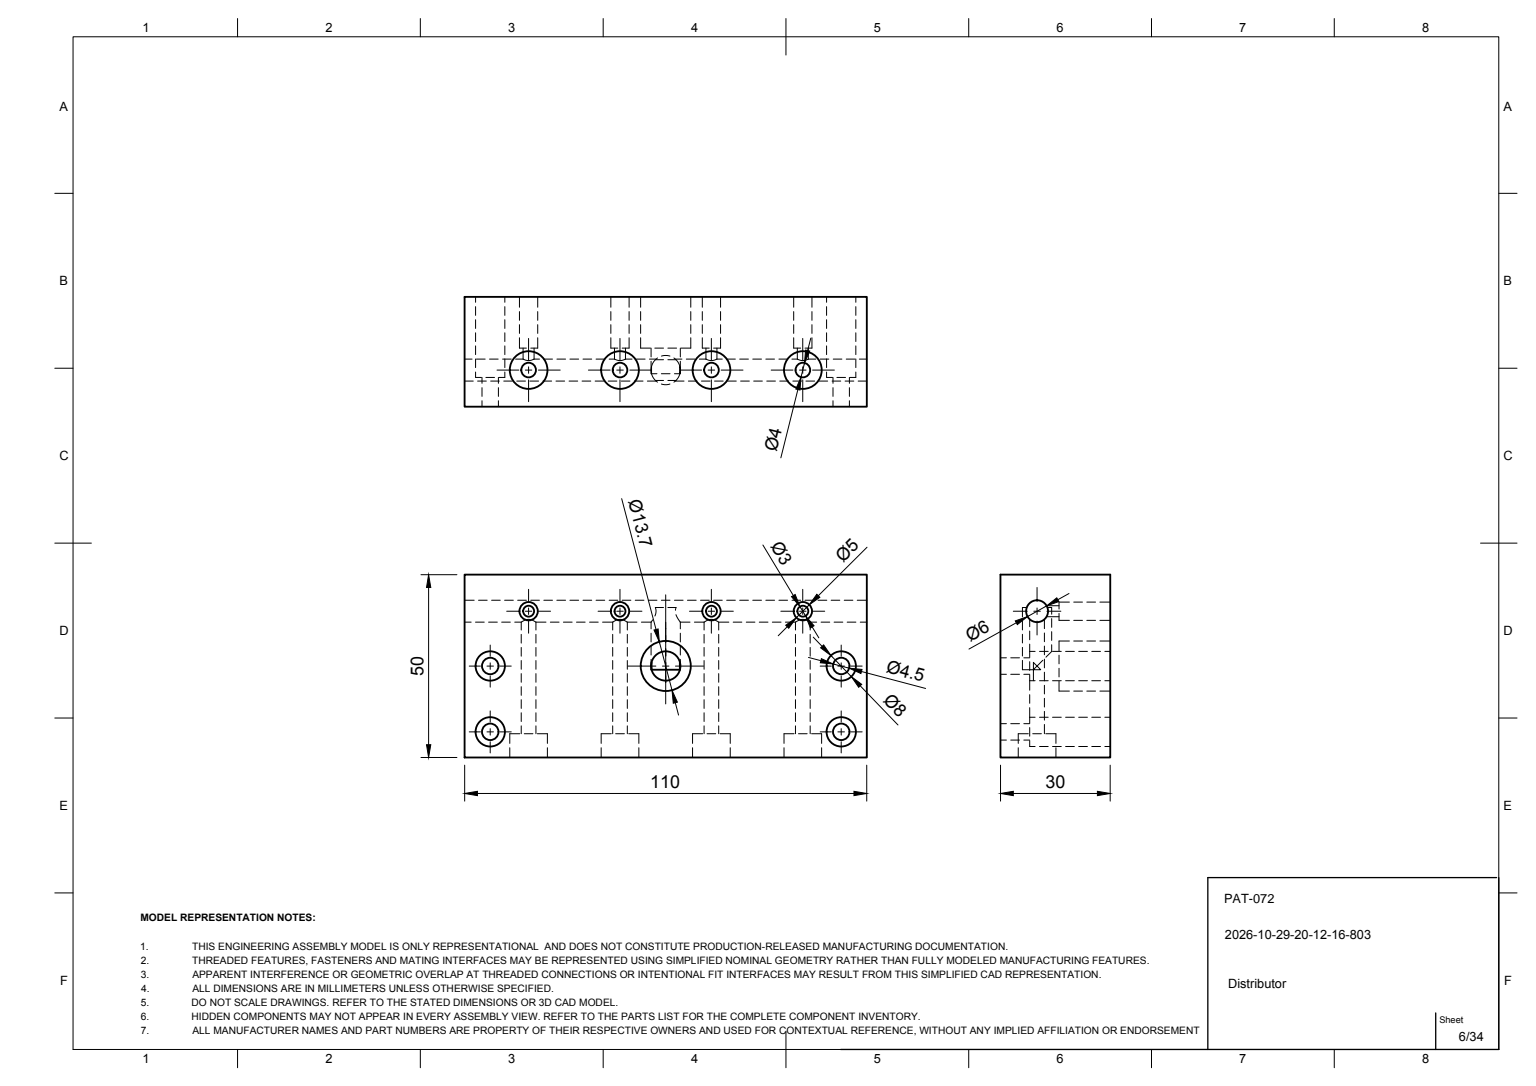
ISO-10303-21;
HEADER;
/* Generated by software containing ST-Developer
 * from STEP Tools, Inc. (www.steptools.com) 
 */

FILE_DESCRIPTION(
/* description */ ('PAT-072'),
/* implementation_level */ '2;1');

FILE_NAME(
/* name */ 'Distributor.step',
/* time_stamp */ '2026-10-29T20:11:56-07:00',
/* author */ (''),
/* organization */ (''),
/* preprocessor_version */ 'ST-DEVELOPER v20.2',
/* originating_system */ 'Autodesk Translation Framework v15.17.0.0',
/* authorisation */ '');

FILE_SCHEMA (('AUTOMOTIVE_DESIGN { 1 0 10303 214 3 1 1 }'));
ENDSEC;

DATA;
#10=MECHANICAL_DESIGN_GEOMETRIC_PRESENTATION_REPRESENTATION('',(#335),#11432);
#224=B_SPLINE_CURVE_WITH_KNOTS('',3,(#9391,#9392,#9393,#9394,#9395,#9396,
#9397,#9398,#9399,#9400,#9401,#9402),.UNSPECIFIED.,.F.,.F.,(4,2,2,2,2,4),
(-0.95677561507049,-0.896341583425282,-0.835907551780073,-0.715039488489656,
-0.596713648012451,-0.478387807535245),.UNSPECIFIED.);
#225=B_SPLINE_CURVE_WITH_KNOTS('',3,(#9403,#9404,#9405,#9406,#9407,#9408),
 .UNSPECIFIED.,.F.,.F.,(4,2,4),(-1.05899336181655,-1.0172096467157,-0.95677561507049),
 .UNSPECIFIED.);
#226=B_SPLINE_CURVE_WITH_KNOTS('',3,(#9410,#9411,#9412,#9413,#9414,#9415),
 .UNSPECIFIED.,.F.,.F.,(4,2,4),(0.95677561507049,1.0172096467157,1.0589933625076),
 .UNSPECIFIED.);
#227=B_SPLINE_CURVE_WITH_KNOTS('',3,(#9417,#9418,#9419,#9420,#9421,#9422,
#9423,#9424,#9425,#9426,#9427,#9428,#9429,#9430,#9431,#9432,#9433,#9434,
#9435,#9436,#9437,#9438,#9439,#9440,#9441,#9442,#9443),.UNSPECIFIED.,.F.,
 .F.,(4,2,3,2,2,2,2,2,2,2,2,2,4),(-0.102217746746057,-0.0604340316452083,
0.,0.0604340316452084,0.120868063290417,0.241736126580834,0.36006196705804,
0.478387807535245,0.596713648012451,0.715039488489657,0.835907551780073,
0.896341583425282,0.95677561507049),.UNSPECIFIED.);
#228=B_SPLINE_CURVE_WITH_KNOTS('',3,(#9446,#9447,#9448,#9449,#9450,#9451,
#9452,#9453,#9454,#9455,#9456,#9457,#9458,#9459,#9460,#9461,#9462),
 .UNSPECIFIED.,.F.,.F.,(4,2,2,2,2,3,2,4),(-0.478387807535245,-0.360061967058039,
-0.241736126580834,-0.120868063290417,-0.0604340316452083,0.,0.0604340316452084,
0.102217747437108),.UNSPECIFIED.);
#229=B_SPLINE_CURVE_WITH_KNOTS('',3,(#9498,#9499,#9500,#9501,#9502,#9503,
#9504,#9505,#9506,#9507),.UNSPECIFIED.,.F.,.F.,(4,2,2,2,4),(0.,0.0577372801322209,
0.115474560264442,0.173054445763352,0.230634331262262),.UNSPECIFIED.);
#230=B_SPLINE_CURVE_WITH_KNOTS('',3,(#9509,#9510,#9511,#9512,#9513,#9514,
#9515,#9516,#9517,#9518),.UNSPECIFIED.,.F.,.F.,(4,2,2,2,4),(0.691902993786785,
0.749482879285695,0.807062764784605,0.864800044916826,0.922537325049047),
 .UNSPECIFIED.);
#231=B_SPLINE_CURVE_WITH_KNOTS('',3,(#9522,#9523,#9524,#9525,#9526,#9527,
#9528,#9529,#9530,#9531,#9532,#9533,#9534,#9535,#9536,#9537,#9538,#9539),
 .UNSPECIFIED.,.F.,.F.,(4,2,2,2,2,2,2,2,4),(0.230634331262262,0.288214216761172,
0.345794102260082,0.403531382392303,0.461268662524523,0.519005942656744,
0.576743222788965,0.634323108287875,0.691902993786785),.UNSPECIFIED.);
#232=B_SPLINE_CURVE_WITH_KNOTS('',3,(#9553,#9554,#9555,#9556,#9557,#9558,
#9559,#9560,#9561,#9562),.UNSPECIFIED.,.F.,.F.,(4,2,2,2,4),(0.,0.07890547039326,
0.15781094078652,0.235848341776528,0.313885742766535),.UNSPECIFIED.);
#233=B_SPLINE_CURVE_WITH_KNOTS('',3,(#9563,#9564,#9565,#9566,#9567,#9568,
#9569,#9570,#9571,#9572,#9573,#9574,#9575,#9576,#9577,#9578,#9579,#9580,
#9581,#9582,#9583,#9584,#9585,#9586,#9587,#9588),.UNSPECIFIED.,.F.,.F.,
(4,2,2,2,2,2,2,2,2,2,2,2,4),(0.313885742766535,0.391923143756543,0.469960544746551,
0.548866015139811,0.627771485533071,0.706676955926331,0.78558242631959,
0.863619827309598,0.941657228299606,1.01969462928961,1.09773203027962,1.17663750067288,
1.25554297106614),.UNSPECIFIED.);
#234=B_SPLINE_CURVE_WITH_KNOTS('',3,(#9599,#9600,#9601,#9602,#9603,#9604,
#9605,#9606,#9607,#9608),.UNSPECIFIED.,.F.,.F.,(4,2,2,2,4),(0.,0.0577372801322209,
0.115474560264442,0.173054445763352,0.230634331262262),.UNSPECIFIED.);
#235=B_SPLINE_CURVE_WITH_KNOTS('',3,(#9610,#9611,#9612,#9613,#9614,#9615,
#9616,#9617,#9618,#9619),.UNSPECIFIED.,.F.,.F.,(4,2,2,2,4),(0.691902993786785,
0.749482879285695,0.807062764784605,0.864800044916825,0.922537325049046),
 .UNSPECIFIED.);
#236=B_SPLINE_CURVE_WITH_KNOTS('',3,(#9623,#9624,#9625,#9626,#9627,#9628,
#9629,#9630,#9631,#9632,#9633,#9634,#9635,#9636,#9637,#9638,#9639,#9640),
 .UNSPECIFIED.,.F.,.F.,(4,2,2,2,2,2,2,2,4),(0.230634331262262,0.288214216761172,
0.345794102260082,0.403531382392303,0.461268662524523,0.519005942656744,
0.576743222788965,0.634323108287875,0.691902993786785),.UNSPECIFIED.);
#237=B_SPLINE_CURVE_WITH_KNOTS('',3,(#9654,#9655,#9656,#9657,#9658,#9659,
#9660,#9661,#9662,#9663),.UNSPECIFIED.,.F.,.F.,(4,2,2,2,4),(0.,0.0789054703932595,
0.157810940786519,0.235848341776527,0.313885742766535),.UNSPECIFIED.);
#238=B_SPLINE_CURVE_WITH_KNOTS('',3,(#9664,#9665,#9666,#9667,#9668,#9669,
#9670,#9671,#9672,#9673,#9674,#9675,#9676,#9677,#9678,#9679,#9680,#9681,
#9682,#9683,#9684,#9685,#9686,#9687,#9688,#9689),.UNSPECIFIED.,.F.,.F.,
(4,2,2,2,2,2,2,2,2,2,2,2,4),(0.313885742766535,0.391923143756543,0.46996054474655,
0.54886601513981,0.627771485533069,0.706676955926329,0.785582426319588,
0.863619827309596,0.941657228299605,1.01969462928961,1.09773203027962,1.17663750067288,
1.25554297106614),.UNSPECIFIED.);
#239=B_SPLINE_CURVE_WITH_KNOTS('',3,(#9700,#9701,#9702,#9703,#9704,#9705,
#9706,#9707,#9708,#9709),.UNSPECIFIED.,.F.,.F.,(4,2,2,2,4),(0.,0.0577372801322209,
0.115474560264442,0.173054445763352,0.230634331262262),.UNSPECIFIED.);
#240=B_SPLINE_CURVE_WITH_KNOTS('',3,(#9711,#9712,#9713,#9714,#9715,#9716,
#9717,#9718,#9719,#9720),.UNSPECIFIED.,.F.,.F.,(4,2,2,2,4),(0.691902993786785,
0.749482879285695,0.807062764784605,0.864800044916826,0.922537325049047),
 .UNSPECIFIED.);
#241=B_SPLINE_CURVE_WITH_KNOTS('',3,(#9724,#9725,#9726,#9727,#9728,#9729,
#9730,#9731,#9732,#9733,#9734,#9735,#9736,#9737,#9738,#9739,#9740,#9741),
 .UNSPECIFIED.,.F.,.F.,(4,2,2,2,2,2,2,2,4),(0.230634331262262,0.288214216761172,
0.345794102260082,0.403531382392303,0.461268662524523,0.519005942656744,
0.576743222788965,0.634323108287875,0.691902993786785),.UNSPECIFIED.);
#242=B_SPLINE_CURVE_WITH_KNOTS('',3,(#9755,#9756,#9757,#9758,#9759,#9760,
#9761,#9762,#9763,#9764),.UNSPECIFIED.,.F.,.F.,(4,2,2,2,4),(0.,0.0789054703932595,
0.157810940786519,0.235848341776527,0.313885742766535),.UNSPECIFIED.);
#243=B_SPLINE_CURVE_WITH_KNOTS('',3,(#9765,#9766,#9767,#9768,#9769,#9770,
#9771,#9772,#9773,#9774,#9775,#9776,#9777,#9778,#9779,#9780,#9781,#9782,
#9783,#9784,#9785,#9786,#9787,#9788,#9789,#9790),.UNSPECIFIED.,.F.,.F.,
(4,2,2,2,2,2,2,2,2,2,2,2,4),(0.313885742766535,0.391923143756543,0.46996054474655,
0.54886601513981,0.627771485533069,0.706676955926329,0.785582426319588,
0.863619827309596,0.941657228299605,1.01969462928961,1.09773203027962,1.17663750067288,
1.25554297106614),.UNSPECIFIED.);
#244=B_SPLINE_CURVE_WITH_KNOTS('',3,(#9801,#9802,#9803,#9804,#9805,#9806,
#9807,#9808,#9809,#9810),.UNSPECIFIED.,.F.,.F.,(4,2,2,2,4),(0.,0.0577372801322209,
0.115474560264442,0.173054445763352,0.230634331262262),.UNSPECIFIED.);
#245=B_SPLINE_CURVE_WITH_KNOTS('',3,(#9812,#9813,#9814,#9815,#9816,#9817,
#9818,#9819,#9820,#9821),.UNSPECIFIED.,.F.,.F.,(4,2,2,2,4),(0.691902993786786,
0.749482879285696,0.807062764784606,0.864800044916827,0.922537325049048),
 .UNSPECIFIED.);
#246=B_SPLINE_CURVE_WITH_KNOTS('',3,(#9825,#9826,#9827,#9828,#9829,#9830,
#9831,#9832,#9833,#9834,#9835,#9836,#9837,#9838,#9839,#9840,#9841,#9842),
 .UNSPECIFIED.,.F.,.F.,(4,2,2,2,2,2,2,2,4),(0.230634331262262,0.288214216761172,
0.345794102260082,0.403531382392303,0.461268662524524,0.519005942656745,
0.576743222788966,0.634323108287876,0.691902993786786),.UNSPECIFIED.);
#247=B_SPLINE_CURVE_WITH_KNOTS('',3,(#9856,#9857,#9858,#9859,#9860,#9861,
#9862,#9863,#9864,#9865),.UNSPECIFIED.,.F.,.F.,(4,2,2,2,4),(0.,0.07890547039326,
0.15781094078652,0.235848341776528,0.313885742766535),.UNSPECIFIED.);
#248=B_SPLINE_CURVE_WITH_KNOTS('',3,(#9866,#9867,#9868,#9869,#9870,#9871,
#9872,#9873,#9874,#9875,#9876,#9877,#9878,#9879,#9880,#9881,#9882,#9883,
#9884,#9885,#9886,#9887,#9888,#9889,#9890,#9891),.UNSPECIFIED.,.F.,.F.,
(4,2,2,2,2,2,2,2,2,2,2,2,4),(0.313885742766535,0.391923143756543,0.469960544746551,
0.548866015139811,0.627771485533071,0.70667695592633,0.78558242631959,0.863619827309598,
0.941657228299606,1.01969462928961,1.09773203027962,1.17663750067288,1.25554297106614),
 .UNSPECIFIED.);
#253=ELLIPSE('',#6580,0.565685424949238,0.4);
#254=ELLIPSE('',#6581,0.565685424949238,0.4);
#255=ELLIPSE('',#6583,0.565685424949238,0.4);
#256=ELLIPSE('',#6585,0.565685424949238,0.4);
#257=ELLIPSE('',#6586,0.565685424949238,0.4);
#258=ELLIPSE('',#6588,0.565685424949238,0.4);
#259=ELLIPSE('',#6590,0.565685424949238,0.4);
#263=SHAPE_REPRESENTATION_RELATIONSHIP('SRR','None',#11567,#299);
#299=ADVANCED_BREP_SHAPE_REPRESENTATION('',(#371),#11398);
#335=STYLED_ITEM('',(#11833),#371);
#371=MANIFOLD_SOLID_BREP('Body1',#6070);
#424=FACE_BOUND('',#1244,.T.);
#425=FACE_BOUND('',#1248,.T.);
#426=FACE_BOUND('',#1252,.T.);
#427=FACE_BOUND('',#1256,.T.);
#428=FACE_BOUND('',#1260,.T.);
#429=FACE_BOUND('',#1264,.T.);
#430=FACE_BOUND('',#1268,.T.);
#431=FACE_BOUND('',#1272,.T.);
#432=FACE_BOUND('',#1276,.T.);
#433=FACE_BOUND('',#1278,.T.);
#434=FACE_BOUND('',#1279,.T.);
#435=FACE_BOUND('',#1280,.T.);
#436=FACE_BOUND('',#1281,.T.);
#437=FACE_BOUND('',#1284,.T.);
#438=FACE_BOUND('',#1287,.T.);
#439=FACE_BOUND('',#1290,.T.);
#440=FACE_BOUND('',#1293,.T.);
#441=FACE_BOUND('',#1300,.T.);
#442=FACE_BOUND('',#1302,.T.);
#443=FACE_BOUND('',#1303,.T.);
#444=FACE_BOUND('',#1304,.T.);
#445=FACE_BOUND('',#1305,.T.);
#446=FACE_BOUND('',#1307,.T.);
#447=FACE_BOUND('',#1309,.T.);
#448=FACE_BOUND('',#1310,.T.);
#449=FACE_BOUND('',#1311,.T.);
#450=FACE_BOUND('',#1312,.T.);
#451=FACE_BOUND('',#1313,.T.);
#452=FACE_BOUND('',#1314,.T.);
#453=FACE_BOUND('',#1315,.T.);
#454=FACE_BOUND('',#1316,.T.);
#455=FACE_BOUND('',#1317,.T.);
#456=FACE_BOUND('',#1319,.T.);
#457=FACE_BOUND('',#1320,.T.);
#458=FACE_BOUND('',#1321,.T.);
#459=FACE_BOUND('',#1322,.T.);
#594=PLANE('',#6573);
#595=PLANE('',#6575);
#596=PLANE('',#6577);
#597=PLANE('',#6591);
#598=PLANE('',#6592);
#599=PLANE('',#6593);
#600=PLANE('',#6595);
#601=PLANE('',#6602);
#602=PLANE('',#6606);
#603=PLANE('',#6612);
#604=PLANE('',#6618);
#605=PLANE('',#6624);
#606=PLANE('',#6630);
#607=PLANE('',#6636);
#608=PLANE('',#6642);
#609=PLANE('',#6648);
#610=PLANE('',#6654);
#611=PLANE('',#6661);
#612=PLANE('',#6666);
#613=PLANE('',#6671);
#614=PLANE('',#6676);
#615=PLANE('',#6686);
#616=PLANE('',#6687);
#617=PLANE('',#6688);
#618=PLANE('',#6689);
#619=PLANE('',#6690);
#620=PLANE('',#6691);
#834=FACE_OUTER_BOUND('',#1228,.T.);
#835=FACE_OUTER_BOUND('',#1229,.T.);
#836=FACE_OUTER_BOUND('',#1230,.T.);
#837=FACE_OUTER_BOUND('',#1231,.T.);
#838=FACE_OUTER_BOUND('',#1232,.T.);
#839=FACE_OUTER_BOUND('',#1233,.T.);
#840=FACE_OUTER_BOUND('',#1234,.T.);
#841=FACE_OUTER_BOUND('',#1235,.T.);
#842=FACE_OUTER_BOUND('',#1236,.T.);
#843=FACE_OUTER_BOUND('',#1237,.T.);
#844=FACE_OUTER_BOUND('',#1238,.T.);
#845=FACE_OUTER_BOUND('',#1239,.T.);
#846=FACE_OUTER_BOUND('',#1240,.T.);
#847=FACE_OUTER_BOUND('',#1241,.T.);
#848=FACE_OUTER_BOUND('',#1242,.T.);
#849=FACE_OUTER_BOUND('',#1243,.T.);
#850=FACE_OUTER_BOUND('',#1245,.T.);
#851=FACE_OUTER_BOUND('',#1246,.T.);
#852=FACE_OUTER_BOUND('',#1247,.T.);
#853=FACE_OUTER_BOUND('',#1249,.T.);
#854=FACE_OUTER_BOUND('',#1250,.T.);
#855=FACE_OUTER_BOUND('',#1251,.T.);
#856=FACE_OUTER_BOUND('',#1253,.T.);
#857=FACE_OUTER_BOUND('',#1254,.T.);
#858=FACE_OUTER_BOUND('',#1255,.T.);
#859=FACE_OUTER_BOUND('',#1257,.T.);
#860=FACE_OUTER_BOUND('',#1258,.T.);
#861=FACE_OUTER_BOUND('',#1259,.T.);
#862=FACE_OUTER_BOUND('',#1261,.T.);
#863=FACE_OUTER_BOUND('',#1262,.T.);
#864=FACE_OUTER_BOUND('',#1263,.T.);
#865=FACE_OUTER_BOUND('',#1265,.T.);
#866=FACE_OUTER_BOUND('',#1266,.T.);
#867=FACE_OUTER_BOUND('',#1267,.T.);
#868=FACE_OUTER_BOUND('',#1269,.T.);
#869=FACE_OUTER_BOUND('',#1270,.T.);
#870=FACE_OUTER_BOUND('',#1271,.T.);
#871=FACE_OUTER_BOUND('',#1273,.T.);
#872=FACE_OUTER_BOUND('',#1274,.T.);
#873=FACE_OUTER_BOUND('',#1275,.T.);
#874=FACE_OUTER_BOUND('',#1277,.T.);
#875=FACE_OUTER_BOUND('',#1282,.T.);
#876=FACE_OUTER_BOUND('',#1283,.T.);
#877=FACE_OUTER_BOUND('',#1285,.T.);
#878=FACE_OUTER_BOUND('',#1286,.T.);
#879=FACE_OUTER_BOUND('',#1288,.T.);
#880=FACE_OUTER_BOUND('',#1289,.T.);
#881=FACE_OUTER_BOUND('',#1291,.T.);
#882=FACE_OUTER_BOUND('',#1292,.T.);
#883=FACE_OUTER_BOUND('',#1294,.T.);
#884=FACE_OUTER_BOUND('',#1295,.T.);
#885=FACE_OUTER_BOUND('',#1296,.T.);
#886=FACE_OUTER_BOUND('',#1297,.T.);
#887=FACE_OUTER_BOUND('',#1298,.T.);
#888=FACE_OUTER_BOUND('',#1299,.T.);
#889=FACE_OUTER_BOUND('',#1301,.T.);
#890=FACE_OUTER_BOUND('',#1306,.T.);
#891=FACE_OUTER_BOUND('',#1308,.T.);
#892=FACE_OUTER_BOUND('',#1318,.T.);
#1228=EDGE_LOOP('',(#4224,#4225));
#1229=EDGE_LOOP('',(#4226,#4227));
#1230=EDGE_LOOP('',(#4228,#4229));
#1231=EDGE_LOOP('',(#4230,#4231,#4232,#4233,#4234,#4235,#4236,#4237,#4238,
#4239,#4240,#4241,#4242,#4243,#4244));
#1232=EDGE_LOOP('',(#4245,#4246,#4247));
#1233=EDGE_LOOP('',(#4248,#4249,#4250));
#1234=EDGE_LOOP('',(#4251,#4252));
#1235=EDGE_LOOP('',(#4253,#4254));
#1236=EDGE_LOOP('',(#4255,#4256));
#1237=EDGE_LOOP('',(#4257,#4258));
#1238=EDGE_LOOP('',(#4259,#4260,#4261));
#1239=EDGE_LOOP('',(#4262,#4263,#4264,#4265,#4266,#4267,#4268,#4269,#4270));
#1240=EDGE_LOOP('',(#4271,#4272,#4273));
#1241=EDGE_LOOP('',(#4274,#4275));
#1242=EDGE_LOOP('',(#4276,#4277,#4278,#4279));
#1243=EDGE_LOOP('',(#4280));
#1244=EDGE_LOOP('',(#4281));
#1245=EDGE_LOOP('',(#4282,#4283,#4284,#4285,#4286,#4287));
#1246=EDGE_LOOP('',(#4288,#4289,#4290,#4291));
#1247=EDGE_LOOP('',(#4292));
#1248=EDGE_LOOP('',(#4293));
#1249=EDGE_LOOP('',(#4294,#4295,#4296,#4297,#4298));
#1250=EDGE_LOOP('',(#4299,#4300,#4301,#4302));
#1251=EDGE_LOOP('',(#4303));
#1252=EDGE_LOOP('',(#4304));
#1253=EDGE_LOOP('',(#4305,#4306,#4307,#4308,#4309,#4310));
#1254=EDGE_LOOP('',(#4311,#4312,#4313,#4314));
#1255=EDGE_LOOP('',(#4315));
#1256=EDGE_LOOP('',(#4316));
#1257=EDGE_LOOP('',(#4317,#4318,#4319,#4320,#4321));
#1258=EDGE_LOOP('',(#4322,#4323,#4324,#4325));
#1259=EDGE_LOOP('',(#4326));
#1260=EDGE_LOOP('',(#4327));
#1261=EDGE_LOOP('',(#4328,#4329,#4330,#4331,#4332,#4333));
#1262=EDGE_LOOP('',(#4334,#4335,#4336,#4337));
#1263=EDGE_LOOP('',(#4338));
#1264=EDGE_LOOP('',(#4339));
#1265=EDGE_LOOP('',(#4340,#4341,#4342,#4343,#4344));
#1266=EDGE_LOOP('',(#4345,#4346,#4347,#4348));
#1267=EDGE_LOOP('',(#4349));
#1268=EDGE_LOOP('',(#4350));
#1269=EDGE_LOOP('',(#4351,#4352,#4353,#4354,#4355,#4356));
#1270=EDGE_LOOP('',(#4357,#4358,#4359,#4360));
#1271=EDGE_LOOP('',(#4361));
#1272=EDGE_LOOP('',(#4362));
#1273=EDGE_LOOP('',(#4363,#4364,#4365,#4366,#4367));
#1274=EDGE_LOOP('',(#4368,#4369,#4370,#4371));
#1275=EDGE_LOOP('',(#4372));
#1276=EDGE_LOOP('',(#4373));
#1277=EDGE_LOOP('',(#4374,#4375,#4376,#4377,#4378,#4379,#4380,#4381,#4382,
#4383,#4384,#4385,#4386,#4387,#4388,#4389,#4390,#4391,#4392,#4393,#4394,
#4395,#4396,#4397,#4398,#4399,#4400,#4401,#4402,#4403,#4404,#4405,#4406));
#1278=EDGE_LOOP('',(#4407,#4408));
#1279=EDGE_LOOP('',(#4409,#4410));
#1280=EDGE_LOOP('',(#4411,#4412));
#1281=EDGE_LOOP('',(#4413,#4414));
#1282=EDGE_LOOP('',(#4415,#4416,#4417,#4418));
#1283=EDGE_LOOP('',(#4419));
#1284=EDGE_LOOP('',(#4420));
#1285=EDGE_LOOP('',(#4421,#4422,#4423,#4424));
#1286=EDGE_LOOP('',(#4425));
#1287=EDGE_LOOP('',(#4426));
#1288=EDGE_LOOP('',(#4427,#4428,#4429,#4430));
#1289=EDGE_LOOP('',(#4431));
#1290=EDGE_LOOP('',(#4432));
#1291=EDGE_LOOP('',(#4433,#4434,#4435,#4436));
#1292=EDGE_LOOP('',(#4437));
#1293=EDGE_LOOP('',(#4438));
#1294=EDGE_LOOP('',(#4439,#4440,#4441,#4442));
#1295=EDGE_LOOP('',(#4443,#4444,#4445,#4446));
#1296=EDGE_LOOP('',(#4447,#4448,#4449,#4450));
#1297=EDGE_LOOP('',(#4451,#4452,#4453,#4454));
#1298=EDGE_LOOP('',(#4455,#4456,#4457,#4458));
#1299=EDGE_LOOP('',(#4459,#4460,#4461,#4462));
#1300=EDGE_LOOP('',(#4463));
#1301=EDGE_LOOP('',(#4464,#4465,#4466,#4467));
#1302=EDGE_LOOP('',(#4468));
#1303=EDGE_LOOP('',(#4469));
#1304=EDGE_LOOP('',(#4470));
#1305=EDGE_LOOP('',(#4471));
#1306=EDGE_LOOP('',(#4472,#4473,#4474,#4475));
#1307=EDGE_LOOP('',(#4476));
#1308=EDGE_LOOP('',(#4477,#4478,#4479,#4480));
#1309=EDGE_LOOP('',(#4481));
#1310=EDGE_LOOP('',(#4482));
#1311=EDGE_LOOP('',(#4483));
#1312=EDGE_LOOP('',(#4484));
#1313=EDGE_LOOP('',(#4485));
#1314=EDGE_LOOP('',(#4486));
#1315=EDGE_LOOP('',(#4487));
#1316=EDGE_LOOP('',(#4488));
#1317=EDGE_LOOP('',(#4489));
#1318=EDGE_LOOP('',(#4490,#4491,#4492,#4493));
#1319=EDGE_LOOP('',(#4494));
#1320=EDGE_LOOP('',(#4495));
#1321=EDGE_LOOP('',(#4496));
#1322=EDGE_LOOP('',(#4497));
#1758=LINE('',#9368,#2177);
#1759=LINE('',#9372,#2178);
#1760=LINE('',#9377,#2179);
#1761=LINE('',#9381,#2180);
#1762=LINE('',#9383,#2181);
#1763=LINE('',#9389,#2182);
#1764=LINE('',#9473,#2183);
#1765=LINE('',#9475,#2184);
#1766=LINE('',#9483,#2185);
#1767=LINE('',#9492,#2186);
#1768=LINE('',#9520,#2187);
#1769=LINE('',#9544,#2188);
#1770=LINE('',#9551,#2189);
#1771=LINE('',#9593,#2190);
#1772=LINE('',#9621,#2191);
#1773=LINE('',#9645,#2192);
#1774=LINE('',#9652,#2193);
#1775=LINE('',#9694,#2194);
#1776=LINE('',#9722,#2195);
#1777=LINE('',#9746,#2196);
#1778=LINE('',#9753,#2197);
#1779=LINE('',#9795,#2198);
#1780=LINE('',#9823,#2199);
#1781=LINE('',#9847,#2200);
#1782=LINE('',#9854,#2201);
#1783=LINE('',#9896,#2202);
#1784=LINE('',#9902,#2203);
#1785=LINE('',#9903,#2204);
#1786=LINE('',#9904,#2205);
#1787=LINE('',#9905,#2206);
#1788=LINE('',#9906,#2207);
#1789=LINE('',#9908,#2208);
#1790=LINE('',#9914,#2209);
#1791=LINE('',#9923,#2210);
#1792=LINE('',#9932,#2211);
#1793=LINE('',#9941,#2212);
#1794=LINE('',#9949,#2213);
#1795=LINE('',#9953,#2214);
#1796=LINE('',#9957,#2215);
#1797=LINE('',#9961,#2216);
#1798=LINE('',#9965,#2217);
#1799=LINE('',#9967,#2218);
#1800=LINE('',#9969,#2219);
#1801=LINE('',#9970,#2220);
#1802=LINE('',#9973,#2221);
#1803=LINE('',#9975,#2222);
#1804=LINE('',#9976,#2223);
#1805=LINE('',#9979,#2224);
#1806=LINE('',#9981,#2225);
#1807=LINE('',#9982,#2226);
#1808=LINE('',#9984,#2227);
#1809=LINE('',#9985,#2228);
#2177=VECTOR('',#7453,1.);
#2178=VECTOR('',#7458,1.);
#2179=VECTOR('',#7463,1.);
#2180=VECTOR('',#7468,1.);
#2181=VECTOR('',#7469,1.);
#2182=VECTOR('',#7474,0.4);
#2183=VECTOR('',#7495,1.);
#2184=VECTOR('',#7498,1.);
#2185=VECTOR('',#7511,0.4);
#2186=VECTOR('',#7524,0.685);
#2187=VECTOR('',#7531,0.15);
#2188=VECTOR('',#7538,0.25);
#2189=VECTOR('',#7547,0.2);
#2190=VECTOR('',#7552,0.515);
#2191=VECTOR('',#7559,0.15);
#2192=VECTOR('',#7566,0.25);
#2193=VECTOR('',#7575,0.2);
#2194=VECTOR('',#7580,0.515);
#2195=VECTOR('',#7587,0.15);
#2196=VECTOR('',#7594,0.25);
#2197=VECTOR('',#7603,0.2);
#2198=VECTOR('',#7608,0.515);
#2199=VECTOR('',#7615,0.15);
#2200=VECTOR('',#7622,0.25);
#2201=VECTOR('',#7631,0.2);
#2202=VECTOR('',#7636,0.515);
#2203=VECTOR('',#7645,0.3);
#2204=VECTOR('',#7646,0.3);
#2205=VECTOR('',#7647,0.3);
#2206=VECTOR('',#7648,0.3);
#2207=VECTOR('',#7649,0.3);
#2208=VECTOR('',#7650,0.3);
#2209=VECTOR('',#7657,0.4);
#2210=VECTOR('',#7668,0.4);
#2211=VECTOR('',#7679,0.4);
#2212=VECTOR('',#7690,0.4);
#2213=VECTOR('',#7701,0.225);
#2214=VECTOR('',#7706,0.225);
#2215=VECTOR('',#7711,0.225);
#2216=VECTOR('',#7716,0.225);
#2217=VECTOR('',#7719,1.);
#2218=VECTOR('',#7720,1.);
#2219=VECTOR('',#7721,1.);
#2220=VECTOR('',#7722,1.);
#2221=VECTOR('',#7725,1.);
#2222=VECTOR('',#7726,1.);
#2223=VECTOR('',#7727,1.);
#2224=VECTOR('',#7730,1.);
#2225=VECTOR('',#7731,1.);
#2226=VECTOR('',#7732,1.);
#2227=VECTOR('',#7735,1.);
#2228=VECTOR('',#7736,1.);
#2574=CIRCLE('',#6574,0.4);
#2575=CIRCLE('',#6576,0.4);
#2576=CIRCLE('',#6578,0.4);
#2577=CIRCLE('',#6582,0.4);
#2578=CIRCLE('',#6589,0.4);
#2579=CIRCLE('',#6594,0.4);
#2580=CIRCLE('',#6596,0.4);
#2581=CIRCLE('',#6599,0.4);
#2582=CIRCLE('',#6601,0.4);
#2583=CIRCLE('',#6604,0.685);
#2584=CIRCLE('',#6605,0.685);
#2585=CIRCLE('',#6608,0.15);
#2586=CIRCLE('',#6610,0.25);
#2587=CIRCLE('',#6611,0.25);
#2588=CIRCLE('',#6614,0.2);
#2589=CIRCLE('',#6616,0.515);
#2590=CIRCLE('',#6617,0.515);
#2591=CIRCLE('',#6620,0.15);
#2592=CIRCLE('',#6622,0.25);
#2593=CIRCLE('',#6623,0.25);
#2594=CIRCLE('',#6626,0.2);
#2595=CIRCLE('',#6628,0.515);
#2596=CIRCLE('',#6629,0.515);
#2597=CIRCLE('',#6632,0.15);
#2598=CIRCLE('',#6634,0.25);
#2599=CIRCLE('',#6635,0.25);
#2600=CIRCLE('',#6638,0.2);
#2601=CIRCLE('',#6640,0.515);
#2602=CIRCLE('',#6641,0.515);
#2603=CIRCLE('',#6644,0.15);
#2604=CIRCLE('',#6646,0.25);
#2605=CIRCLE('',#6647,0.25);
#2606=CIRCLE('',#6650,0.2);
#2607=CIRCLE('',#6652,0.515);
#2608=CIRCLE('',#6653,0.515);
#2609=CIRCLE('',#6656,0.3);
#2610=CIRCLE('',#6657,0.3);
#2611=CIRCLE('',#6659,0.4);
#2612=CIRCLE('',#6660,0.4);
#2613=CIRCLE('',#6662,0.225);
#2614=CIRCLE('',#6664,0.4);
#2615=CIRCLE('',#6665,0.4);
#2616=CIRCLE('',#6667,0.225);
#2617=CIRCLE('',#6669,0.4);
#2618=CIRCLE('',#6670,0.4);
#2619=CIRCLE('',#6672,0.225);
#2620=CIRCLE('',#6674,0.4);
#2621=CIRCLE('',#6675,0.4);
#2622=CIRCLE('',#6677,0.225);
#2623=CIRCLE('',#6679,0.225);
#2624=CIRCLE('',#6681,0.225);
#2625=CIRCLE('',#6683,0.225);
#2626=CIRCLE('',#6685,0.225);
#2888=VERTEX_POINT('',#9366);
#2889=VERTEX_POINT('',#9367);
#2890=VERTEX_POINT('',#9371);
#2891=VERTEX_POINT('',#9375);
#2892=VERTEX_POINT('',#9376);
#2893=VERTEX_POINT('',#9380);
#2894=VERTEX_POINT('',#9382);
#2895=VERTEX_POINT('',#9384);
#2896=VERTEX_POINT('',#9386);
#2897=VERTEX_POINT('',#9388);
#2898=VERTEX_POINT('',#9390);
#2899=VERTEX_POINT('',#9409);
#2900=VERTEX_POINT('',#9416);
#2901=VERTEX_POINT('',#9444);
#2902=VERTEX_POINT('',#9468);
#2903=VERTEX_POINT('',#9482);
#2904=VERTEX_POINT('',#9489);
#2905=VERTEX_POINT('',#9491);
#2906=VERTEX_POINT('',#9496);
#2907=VERTEX_POINT('',#9497);
#2908=VERTEX_POINT('',#9508);
#2909=VERTEX_POINT('',#9519);
#2910=VERTEX_POINT('',#9541);
#2911=VERTEX_POINT('',#9543);
#2912=VERTEX_POINT('',#9548);
#2913=VERTEX_POINT('',#9550);
#2914=VERTEX_POINT('',#9552);
#2915=VERTEX_POINT('',#9590);
#2916=VERTEX_POINT('',#9592);
#2917=VERTEX_POINT('',#9597);
#2918=VERTEX_POINT('',#9598);
#2919=VERTEX_POINT('',#9609);
#2920=VERTEX_POINT('',#9620);
#2921=VERTEX_POINT('',#9642);
#2922=VERTEX_POINT('',#9644);
#2923=VERTEX_POINT('',#9649);
#2924=VERTEX_POINT('',#9651);
#2925=VERTEX_POINT('',#9653);
#2926=VERTEX_POINT('',#9691);
#2927=VERTEX_POINT('',#9693);
#2928=VERTEX_POINT('',#9698);
#2929=VERTEX_POINT('',#9699);
#2930=VERTEX_POINT('',#9710);
#2931=VERTEX_POINT('',#9721);
#2932=VERTEX_POINT('',#9743);
#2933=VERTEX_POINT('',#9745);
#2934=VERTEX_POINT('',#9750);
#2935=VERTEX_POINT('',#9752);
#2936=VERTEX_POINT('',#9754);
#2937=VERTEX_POINT('',#9792);
#2938=VERTEX_POINT('',#9794);
#2939=VERTEX_POINT('',#9799);
#2940=VERTEX_POINT('',#9800);
#2941=VERTEX_POINT('',#9811);
#2942=VERTEX_POINT('',#9822);
#2943=VERTEX_POINT('',#9844);
#2944=VERTEX_POINT('',#9846);
#2945=VERTEX_POINT('',#9851);
#2946=VERTEX_POINT('',#9853);
#2947=VERTEX_POINT('',#9855);
#2948=VERTEX_POINT('',#9893);
#2949=VERTEX_POINT('',#9895);
#2950=VERTEX_POINT('',#9900);
#2951=VERTEX_POINT('',#9907);
#2952=VERTEX_POINT('',#9911);
#2953=VERTEX_POINT('',#9913);
#2954=VERTEX_POINT('',#9917);
#2955=VERTEX_POINT('',#9920);
#2956=VERTEX_POINT('',#9922);
#2957=VERTEX_POINT('',#9926);
#2958=VERTEX_POINT('',#9929);
#2959=VERTEX_POINT('',#9931);
#2960=VERTEX_POINT('',#9935);
#2961=VERTEX_POINT('',#9938);
#2962=VERTEX_POINT('',#9940);
#2963=VERTEX_POINT('',#9944);
#2964=VERTEX_POINT('',#9947);
#2965=VERTEX_POINT('',#9951);
#2966=VERTEX_POINT('',#9955);
#2967=VERTEX_POINT('',#9959);
#2968=VERTEX_POINT('',#9963);
#2969=VERTEX_POINT('',#9964);
#2970=VERTEX_POINT('',#9966);
#2971=VERTEX_POINT('',#9968);
#2972=VERTEX_POINT('',#9972);
#2973=VERTEX_POINT('',#9974);
#2974=VERTEX_POINT('',#9978);
#2975=VERTEX_POINT('',#9980);
#3401=EDGE_CURVE('',#2888,#2889,#1758,.T.);
#3402=EDGE_CURVE('',#2888,#2889,#2574,.T.);
#3403=EDGE_CURVE('',#2890,#2888,#1759,.T.);
#3404=EDGE_CURVE('',#2890,#2888,#2575,.T.);
#3405=EDGE_CURVE('',#2891,#2892,#1760,.T.);
#3406=EDGE_CURVE('',#2892,#2891,#2576,.T.);
#3407=EDGE_CURVE('',#2889,#2893,#1761,.T.);
#3408=EDGE_CURVE('',#2894,#2888,#1762,.T.);
#3409=EDGE_CURVE('',#2895,#2894,#253,.T.);
#3410=EDGE_CURVE('',#2896,#2895,#254,.T.);
#3411=EDGE_CURVE('',#2896,#2897,#1763,.T.);
#3412=EDGE_CURVE('',#2898,#2897,#224,.T.);
#3413=EDGE_CURVE('',#2892,#2898,#225,.T.);
#3414=EDGE_CURVE('',#2899,#2891,#226,.T.);
#3415=EDGE_CURVE('',#2900,#2899,#227,.T.);
#3416=EDGE_CURVE('',#2900,#2901,#2577,.T.);
#3417=EDGE_CURVE('',#2897,#2901,#228,.T.);
#3418=EDGE_CURVE('',#2893,#2896,#255,.T.);
#3419=EDGE_CURVE('',#2895,#2890,#256,.T.);
#3420=EDGE_CURVE('',#2888,#2895,#257,.T.);
#3421=EDGE_CURVE('',#2902,#2896,#258,.T.);
#3422=EDGE_CURVE('',#2889,#2902,#2578,.T.);
#3423=EDGE_CURVE('',#2896,#2889,#259,.T.);
#3424=EDGE_CURVE('',#2901,#2900,#1764,.T.);
#3425=EDGE_CURVE('',#2889,#2902,#1765,.T.);
#3426=EDGE_CURVE('',#2888,#2894,#2579,.T.);
#3427=EDGE_CURVE('',#2889,#2888,#2580,.T.);
#3428=EDGE_CURVE('',#2896,#2903,#1766,.T.);
#3429=EDGE_CURVE('',#2903,#2903,#2581,.T.);
#3430=EDGE_CURVE('',#2893,#2889,#2582,.T.);
#3431=EDGE_CURVE('',#2904,#2904,#2583,.T.);
#3432=EDGE_CURVE('',#2904,#2905,#1767,.T.);
#3433=EDGE_CURVE('',#2905,#2905,#2584,.T.);
#3434=EDGE_CURVE('',#2906,#2907,#229,.T.);
#3435=EDGE_CURVE('',#2908,#2906,#230,.T.);
#3436=EDGE_CURVE('',#2908,#2909,#1768,.T.);
#3437=EDGE_CURVE('',#2909,#2909,#2585,.T.);
#3438=EDGE_CURVE('',#2907,#2908,#231,.T.);
#3439=EDGE_CURVE('',#2910,#2910,#2586,.T.);
#3440=EDGE_CURVE('',#2910,#2911,#1769,.T.);
#3441=EDGE_CURVE('',#2911,#2911,#2587,.T.);
#3442=EDGE_CURVE('',#2912,#2912,#2588,.T.);
#3443=EDGE_CURVE('',#2912,#2913,#1770,.T.);
#3444=EDGE_CURVE('',#2914,#2913,#232,.T.);
#3445=EDGE_CURVE('',#2913,#2914,#233,.T.);
#3446=EDGE_CURVE('',#2915,#2915,#2589,.T.);
#3447=EDGE_CURVE('',#2915,#2916,#1771,.T.);
#3448=EDGE_CURVE('',#2916,#2916,#2590,.T.);
#3449=EDGE_CURVE('',#2917,#2918,#234,.T.);
#3450=EDGE_CURVE('',#2919,#2917,#235,.T.);
#3451=EDGE_CURVE('',#2919,#2920,#1772,.T.);
#3452=EDGE_CURVE('',#2920,#2920,#2591,.T.);
#3453=EDGE_CURVE('',#2918,#2919,#236,.T.);
#3454=EDGE_CURVE('',#2921,#2921,#2592,.T.);
#3455=EDGE_CURVE('',#2921,#2922,#1773,.T.);
#3456=EDGE_CURVE('',#2922,#2922,#2593,.T.);
#3457=EDGE_CURVE('',#2923,#2923,#2594,.T.);
#3458=EDGE_CURVE('',#2923,#2924,#1774,.T.);
#3459=EDGE_CURVE('',#2925,#2924,#237,.T.);
#3460=EDGE_CURVE('',#2924,#2925,#238,.T.);
#3461=EDGE_CURVE('',#2926,#2926,#2595,.T.);
#3462=EDGE_CURVE('',#2926,#2927,#1775,.T.);
#3463=EDGE_CURVE('',#2927,#2927,#2596,.T.);
#3464=EDGE_CURVE('',#2928,#2929,#239,.T.);
#3465=EDGE_CURVE('',#2930,#2928,#240,.T.);
#3466=EDGE_CURVE('',#2930,#2931,#1776,.T.);
#3467=EDGE_CURVE('',#2931,#2931,#2597,.T.);
#3468=EDGE_CURVE('',#2929,#2930,#241,.T.);
#3469=EDGE_CURVE('',#2932,#2932,#2598,.T.);
#3470=EDGE_CURVE('',#2932,#2933,#1777,.T.);
#3471=EDGE_CURVE('',#2933,#2933,#2599,.T.);
#3472=EDGE_CURVE('',#2934,#2934,#2600,.T.);
#3473=EDGE_CURVE('',#2934,#2935,#1778,.T.);
#3474=EDGE_CURVE('',#2936,#2935,#242,.T.);
#3475=EDGE_CURVE('',#2935,#2936,#243,.T.);
#3476=EDGE_CURVE('',#2937,#2937,#2601,.T.);
#3477=EDGE_CURVE('',#2937,#2938,#1779,.T.);
#3478=EDGE_CURVE('',#2938,#2938,#2602,.T.);
#3479=EDGE_CURVE('',#2939,#2940,#244,.T.);
#3480=EDGE_CURVE('',#2941,#2939,#245,.T.);
#3481=EDGE_CURVE('',#2941,#2942,#1780,.T.);
#3482=EDGE_CURVE('',#2942,#2942,#2603,.T.);
#3483=EDGE_CURVE('',#2940,#2941,#246,.T.);
#3484=EDGE_CURVE('',#2943,#2943,#2604,.T.);
#3485=EDGE_CURVE('',#2943,#2944,#1781,.T.);
#3486=EDGE_CURVE('',#2944,#2944,#2605,.T.);
#3487=EDGE_CURVE('',#2945,#2945,#2606,.T.);
#3488=EDGE_CURVE('',#2945,#2946,#1782,.T.);
#3489=EDGE_CURVE('',#2947,#2946,#247,.T.);
#3490=EDGE_CURVE('',#2946,#2947,#248,.T.);
#3491=EDGE_CURVE('',#2948,#2948,#2607,.T.);
#3492=EDGE_CURVE('',#2948,#2949,#1783,.T.);
#3493=EDGE_CURVE('',#2949,#2949,#2608,.T.);
#3494=EDGE_CURVE('',#2950,#2950,#2609,.T.);
#3495=EDGE_CURVE('',#2950,#2941,#1784,.T.);
#3496=EDGE_CURVE('',#2940,#2930,#1785,.T.);
#3497=EDGE_CURVE('',#2929,#2898,#1786,.T.);
#3498=EDGE_CURVE('',#2899,#2919,#1787,.T.);
#3499=EDGE_CURVE('',#2918,#2908,#1788,.T.);
#3500=EDGE_CURVE('',#2907,#2951,#1789,.T.);
#3501=EDGE_CURVE('',#2951,#2951,#2610,.T.);
#3502=EDGE_CURVE('',#2952,#2952,#2611,.T.);
#3503=EDGE_CURVE('',#2952,#2953,#1790,.T.);
#3504=EDGE_CURVE('',#2953,#2953,#2612,.T.);
#3505=EDGE_CURVE('',#2954,#2954,#2613,.T.);
#3506=EDGE_CURVE('',#2955,#2955,#2614,.T.);
#3507=EDGE_CURVE('',#2955,#2956,#1791,.T.);
#3508=EDGE_CURVE('',#2956,#2956,#2615,.T.);
#3509=EDGE_CURVE('',#2957,#2957,#2616,.T.);
#3510=EDGE_CURVE('',#2958,#2958,#2617,.T.);
#3511=EDGE_CURVE('',#2958,#2959,#1792,.T.);
#3512=EDGE_CURVE('',#2959,#2959,#2618,.T.);
#3513=EDGE_CURVE('',#2960,#2960,#2619,.T.);
#3514=EDGE_CURVE('',#2961,#2961,#2620,.T.);
#3515=EDGE_CURVE('',#2961,#2962,#1793,.T.);
#3516=EDGE_CURVE('',#2962,#2962,#2621,.T.);
#3517=EDGE_CURVE('',#2963,#2963,#2622,.T.);
#3518=EDGE_CURVE('',#2964,#2964,#2623,.T.);
#3519=EDGE_CURVE('',#2964,#2954,#1794,.T.);
#3520=EDGE_CURVE('',#2965,#2965,#2624,.T.);
#3521=EDGE_CURVE('',#2965,#2957,#1795,.T.);
#3522=EDGE_CURVE('',#2966,#2966,#2625,.T.);
#3523=EDGE_CURVE('',#2966,#2960,#1796,.T.);
#3524=EDGE_CURVE('',#2967,#2967,#2626,.T.);
#3525=EDGE_CURVE('',#2967,#2963,#1797,.T.);
#3526=EDGE_CURVE('',#2968,#2969,#1798,.T.);
#3527=EDGE_CURVE('',#2969,#2970,#1799,.T.);
#3528=EDGE_CURVE('',#2971,#2970,#1800,.T.);
#3529=EDGE_CURVE('',#2968,#2971,#1801,.T.);
#3530=EDGE_CURVE('',#2972,#2968,#1802,.T.);
#3531=EDGE_CURVE('',#2973,#2971,#1803,.T.);
#3532=EDGE_CURVE('',#2972,#2973,#1804,.T.);
#3533=EDGE_CURVE('',#2974,#2972,#1805,.T.);
#3534=EDGE_CURVE('',#2975,#2973,#1806,.T.);
#3535=EDGE_CURVE('',#2974,#2975,#1807,.T.);
#3536=EDGE_CURVE('',#2969,#2974,#1808,.T.);
#3537=EDGE_CURVE('',#2970,#2975,#1809,.T.);
#4224=ORIENTED_EDGE('',*,*,#3401,.F.);
#4225=ORIENTED_EDGE('',*,*,#3402,.T.);
#4226=ORIENTED_EDGE('',*,*,#3403,.F.);
#4227=ORIENTED_EDGE('',*,*,#3404,.T.);
#4228=ORIENTED_EDGE('',*,*,#3405,.F.);
#4229=ORIENTED_EDGE('',*,*,#3406,.F.);
#4230=ORIENTED_EDGE('',*,*,#3407,.F.);
#4231=ORIENTED_EDGE('',*,*,#3402,.F.);
#4232=ORIENTED_EDGE('',*,*,#3408,.F.);
#4233=ORIENTED_EDGE('',*,*,#3409,.F.);
#4234=ORIENTED_EDGE('',*,*,#3410,.F.);
#4235=ORIENTED_EDGE('',*,*,#3411,.T.);
#4236=ORIENTED_EDGE('',*,*,#3412,.F.);
#4237=ORIENTED_EDGE('',*,*,#3413,.F.);
#4238=ORIENTED_EDGE('',*,*,#3406,.T.);
#4239=ORIENTED_EDGE('',*,*,#3414,.F.);
#4240=ORIENTED_EDGE('',*,*,#3415,.F.);
#4241=ORIENTED_EDGE('',*,*,#3416,.T.);
#4242=ORIENTED_EDGE('',*,*,#3417,.F.);
#4243=ORIENTED_EDGE('',*,*,#3411,.F.);
#4244=ORIENTED_EDGE('',*,*,#3418,.F.);
#4245=ORIENTED_EDGE('',*,*,#3419,.F.);
#4246=ORIENTED_EDGE('',*,*,#3420,.F.);
#4247=ORIENTED_EDGE('',*,*,#3404,.F.);
#4248=ORIENTED_EDGE('',*,*,#3421,.F.);
#4249=ORIENTED_EDGE('',*,*,#3422,.F.);
#4250=ORIENTED_EDGE('',*,*,#3423,.F.);
#4251=ORIENTED_EDGE('',*,*,#3424,.F.);
#4252=ORIENTED_EDGE('',*,*,#3416,.F.);
#4253=ORIENTED_EDGE('',*,*,#3425,.F.);
#4254=ORIENTED_EDGE('',*,*,#3422,.T.);
#4255=ORIENTED_EDGE('',*,*,#3408,.T.);
#4256=ORIENTED_EDGE('',*,*,#3426,.T.);
#4257=ORIENTED_EDGE('',*,*,#3401,.T.);
#4258=ORIENTED_EDGE('',*,*,#3427,.T.);
#4259=ORIENTED_EDGE('',*,*,#3409,.T.);
#4260=ORIENTED_EDGE('',*,*,#3426,.F.);
#4261=ORIENTED_EDGE('',*,*,#3420,.T.);
#4262=ORIENTED_EDGE('',*,*,#3425,.T.);
#4263=ORIENTED_EDGE('',*,*,#3421,.T.);
#4264=ORIENTED_EDGE('',*,*,#3428,.T.);
#4265=ORIENTED_EDGE('',*,*,#3429,.F.);
#4266=ORIENTED_EDGE('',*,*,#3428,.F.);
#4267=ORIENTED_EDGE('',*,*,#3410,.T.);
#4268=ORIENTED_EDGE('',*,*,#3419,.T.);
#4269=ORIENTED_EDGE('',*,*,#3403,.T.);
#4270=ORIENTED_EDGE('',*,*,#3427,.F.);
#4271=ORIENTED_EDGE('',*,*,#3418,.T.);
#4272=ORIENTED_EDGE('',*,*,#3423,.T.);
#4273=ORIENTED_EDGE('',*,*,#3430,.F.);
#4274=ORIENTED_EDGE('',*,*,#3407,.T.);
#4275=ORIENTED_EDGE('',*,*,#3430,.T.);
#4276=ORIENTED_EDGE('',*,*,#3431,.F.);
#4277=ORIENTED_EDGE('',*,*,#3432,.T.);
#4278=ORIENTED_EDGE('',*,*,#3433,.F.);
#4279=ORIENTED_EDGE('',*,*,#3432,.F.);
#4280=ORIENTED_EDGE('',*,*,#3431,.T.);
#4281=ORIENTED_EDGE('',*,*,#3429,.T.);
#4282=ORIENTED_EDGE('',*,*,#3434,.F.);
#4283=ORIENTED_EDGE('',*,*,#3435,.F.);
#4284=ORIENTED_EDGE('',*,*,#3436,.T.);
#4285=ORIENTED_EDGE('',*,*,#3437,.F.);
#4286=ORIENTED_EDGE('',*,*,#3436,.F.);
#4287=ORIENTED_EDGE('',*,*,#3438,.F.);
#4288=ORIENTED_EDGE('',*,*,#3439,.F.);
#4289=ORIENTED_EDGE('',*,*,#3440,.T.);
#4290=ORIENTED_EDGE('',*,*,#3441,.F.);
#4291=ORIENTED_EDGE('',*,*,#3440,.F.);
#4292=ORIENTED_EDGE('',*,*,#3439,.T.);
#4293=ORIENTED_EDGE('',*,*,#3437,.T.);
#4294=ORIENTED_EDGE('',*,*,#3442,.F.);
#4295=ORIENTED_EDGE('',*,*,#3443,.T.);
#4296=ORIENTED_EDGE('',*,*,#3444,.F.);
#4297=ORIENTED_EDGE('',*,*,#3445,.F.);
#4298=ORIENTED_EDGE('',*,*,#3443,.F.);
#4299=ORIENTED_EDGE('',*,*,#3446,.F.);
#4300=ORIENTED_EDGE('',*,*,#3447,.T.);
#4301=ORIENTED_EDGE('',*,*,#3448,.T.);
#4302=ORIENTED_EDGE('',*,*,#3447,.F.);
#4303=ORIENTED_EDGE('',*,*,#3448,.F.);
#4304=ORIENTED_EDGE('',*,*,#3442,.T.);
#4305=ORIENTED_EDGE('',*,*,#3449,.F.);
#4306=ORIENTED_EDGE('',*,*,#3450,.F.);
#4307=ORIENTED_EDGE('',*,*,#3451,.T.);
#4308=ORIENTED_EDGE('',*,*,#3452,.F.);
#4309=ORIENTED_EDGE('',*,*,#3451,.F.);
#4310=ORIENTED_EDGE('',*,*,#3453,.F.);
#4311=ORIENTED_EDGE('',*,*,#3454,.F.);
#4312=ORIENTED_EDGE('',*,*,#3455,.T.);
#4313=ORIENTED_EDGE('',*,*,#3456,.F.);
#4314=ORIENTED_EDGE('',*,*,#3455,.F.);
#4315=ORIENTED_EDGE('',*,*,#3454,.T.);
#4316=ORIENTED_EDGE('',*,*,#3452,.T.);
#4317=ORIENTED_EDGE('',*,*,#3457,.F.);
#4318=ORIENTED_EDGE('',*,*,#3458,.T.);
#4319=ORIENTED_EDGE('',*,*,#3459,.F.);
#4320=ORIENTED_EDGE('',*,*,#3460,.F.);
#4321=ORIENTED_EDGE('',*,*,#3458,.F.);
#4322=ORIENTED_EDGE('',*,*,#3461,.F.);
#4323=ORIENTED_EDGE('',*,*,#3462,.T.);
#4324=ORIENTED_EDGE('',*,*,#3463,.T.);
#4325=ORIENTED_EDGE('',*,*,#3462,.F.);
#4326=ORIENTED_EDGE('',*,*,#3463,.F.);
#4327=ORIENTED_EDGE('',*,*,#3457,.T.);
#4328=ORIENTED_EDGE('',*,*,#3464,.F.);
#4329=ORIENTED_EDGE('',*,*,#3465,.F.);
#4330=ORIENTED_EDGE('',*,*,#3466,.T.);
#4331=ORIENTED_EDGE('',*,*,#3467,.F.);
#4332=ORIENTED_EDGE('',*,*,#3466,.F.);
#4333=ORIENTED_EDGE('',*,*,#3468,.F.);
#4334=ORIENTED_EDGE('',*,*,#3469,.F.);
#4335=ORIENTED_EDGE('',*,*,#3470,.T.);
#4336=ORIENTED_EDGE('',*,*,#3471,.F.);
#4337=ORIENTED_EDGE('',*,*,#3470,.F.);
#4338=ORIENTED_EDGE('',*,*,#3469,.T.);
#4339=ORIENTED_EDGE('',*,*,#3467,.T.);
#4340=ORIENTED_EDGE('',*,*,#3472,.F.);
#4341=ORIENTED_EDGE('',*,*,#3473,.T.);
#4342=ORIENTED_EDGE('',*,*,#3474,.F.);
#4343=ORIENTED_EDGE('',*,*,#3475,.F.);
#4344=ORIENTED_EDGE('',*,*,#3473,.F.);
#4345=ORIENTED_EDGE('',*,*,#3476,.F.);
#4346=ORIENTED_EDGE('',*,*,#3477,.T.);
#4347=ORIENTED_EDGE('',*,*,#3478,.T.);
#4348=ORIENTED_EDGE('',*,*,#3477,.F.);
#4349=ORIENTED_EDGE('',*,*,#3478,.F.);
#4350=ORIENTED_EDGE('',*,*,#3472,.T.);
#4351=ORIENTED_EDGE('',*,*,#3479,.F.);
#4352=ORIENTED_EDGE('',*,*,#3480,.F.);
#4353=ORIENTED_EDGE('',*,*,#3481,.T.);
#4354=ORIENTED_EDGE('',*,*,#3482,.F.);
#4355=ORIENTED_EDGE('',*,*,#3481,.F.);
#4356=ORIENTED_EDGE('',*,*,#3483,.F.);
#4357=ORIENTED_EDGE('',*,*,#3484,.F.);
#4358=ORIENTED_EDGE('',*,*,#3485,.T.);
#4359=ORIENTED_EDGE('',*,*,#3486,.F.);
#4360=ORIENTED_EDGE('',*,*,#3485,.F.);
#4361=ORIENTED_EDGE('',*,*,#3484,.T.);
#4362=ORIENTED_EDGE('',*,*,#3482,.T.);
#4363=ORIENTED_EDGE('',*,*,#3487,.F.);
#4364=ORIENTED_EDGE('',*,*,#3488,.T.);
#4365=ORIENTED_EDGE('',*,*,#3489,.F.);
#4366=ORIENTED_EDGE('',*,*,#3490,.F.);
#4367=ORIENTED_EDGE('',*,*,#3488,.F.);
#4368=ORIENTED_EDGE('',*,*,#3491,.F.);
#4369=ORIENTED_EDGE('',*,*,#3492,.T.);
#4370=ORIENTED_EDGE('',*,*,#3493,.T.);
#4371=ORIENTED_EDGE('',*,*,#3492,.F.);
#4372=ORIENTED_EDGE('',*,*,#3493,.F.);
#4373=ORIENTED_EDGE('',*,*,#3487,.T.);
#4374=ORIENTED_EDGE('',*,*,#3494,.F.);
#4375=ORIENTED_EDGE('',*,*,#3495,.T.);
#4376=ORIENTED_EDGE('',*,*,#3480,.T.);
#4377=ORIENTED_EDGE('',*,*,#3479,.T.);
#4378=ORIENTED_EDGE('',*,*,#3496,.T.);
#4379=ORIENTED_EDGE('',*,*,#3465,.T.);
#4380=ORIENTED_EDGE('',*,*,#3464,.T.);
#4381=ORIENTED_EDGE('',*,*,#3497,.T.);
#4382=ORIENTED_EDGE('',*,*,#3412,.T.);
#4383=ORIENTED_EDGE('',*,*,#3417,.T.);
#4384=ORIENTED_EDGE('',*,*,#3424,.T.);
#4385=ORIENTED_EDGE('',*,*,#3415,.T.);
#4386=ORIENTED_EDGE('',*,*,#3498,.T.);
#4387=ORIENTED_EDGE('',*,*,#3450,.T.);
#4388=ORIENTED_EDGE('',*,*,#3449,.T.);
#4389=ORIENTED_EDGE('',*,*,#3499,.T.);
#4390=ORIENTED_EDGE('',*,*,#3435,.T.);
#4391=ORIENTED_EDGE('',*,*,#3434,.T.);
#4392=ORIENTED_EDGE('',*,*,#3500,.T.);
#4393=ORIENTED_EDGE('',*,*,#3501,.F.);
#4394=ORIENTED_EDGE('',*,*,#3500,.F.);
#4395=ORIENTED_EDGE('',*,*,#3438,.T.);
#4396=ORIENTED_EDGE('',*,*,#3499,.F.);
#4397=ORIENTED_EDGE('',*,*,#3453,.T.);
#4398=ORIENTED_EDGE('',*,*,#3498,.F.);
#4399=ORIENTED_EDGE('',*,*,#3414,.T.);
#4400=ORIENTED_EDGE('',*,*,#3405,.T.);
#4401=ORIENTED_EDGE('',*,*,#3413,.T.);
#4402=ORIENTED_EDGE('',*,*,#3497,.F.);
#4403=ORIENTED_EDGE('',*,*,#3468,.T.);
#4404=ORIENTED_EDGE('',*,*,#3496,.F.);
#4405=ORIENTED_EDGE('',*,*,#3483,.T.);
#4406=ORIENTED_EDGE('',*,*,#3495,.F.);
#4407=ORIENTED_EDGE('',*,*,#3444,.T.);
#4408=ORIENTED_EDGE('',*,*,#3445,.T.);
#4409=ORIENTED_EDGE('',*,*,#3459,.T.);
#4410=ORIENTED_EDGE('',*,*,#3460,.T.);
#4411=ORIENTED_EDGE('',*,*,#3474,.T.);
#4412=ORIENTED_EDGE('',*,*,#3475,.T.);
#4413=ORIENTED_EDGE('',*,*,#3489,.T.);
#4414=ORIENTED_EDGE('',*,*,#3490,.T.);
#4415=ORIENTED_EDGE('',*,*,#3502,.F.);
#4416=ORIENTED_EDGE('',*,*,#3503,.T.);
#4417=ORIENTED_EDGE('',*,*,#3504,.F.);
#4418=ORIENTED_EDGE('',*,*,#3503,.F.);
#4419=ORIENTED_EDGE('',*,*,#3502,.T.);
#4420=ORIENTED_EDGE('',*,*,#3505,.F.);
#4421=ORIENTED_EDGE('',*,*,#3506,.F.);
#4422=ORIENTED_EDGE('',*,*,#3507,.T.);
#4423=ORIENTED_EDGE('',*,*,#3508,.F.);
#4424=ORIENTED_EDGE('',*,*,#3507,.F.);
#4425=ORIENTED_EDGE('',*,*,#3506,.T.);
#4426=ORIENTED_EDGE('',*,*,#3509,.F.);
#4427=ORIENTED_EDGE('',*,*,#3510,.F.);
#4428=ORIENTED_EDGE('',*,*,#3511,.T.);
#4429=ORIENTED_EDGE('',*,*,#3512,.F.);
#4430=ORIENTED_EDGE('',*,*,#3511,.F.);
#4431=ORIENTED_EDGE('',*,*,#3510,.T.);
#4432=ORIENTED_EDGE('',*,*,#3513,.F.);
#4433=ORIENTED_EDGE('',*,*,#3514,.F.);
#4434=ORIENTED_EDGE('',*,*,#3515,.T.);
#4435=ORIENTED_EDGE('',*,*,#3516,.F.);
#4436=ORIENTED_EDGE('',*,*,#3515,.F.);
#4437=ORIENTED_EDGE('',*,*,#3514,.T.);
#4438=ORIENTED_EDGE('',*,*,#3517,.F.);
#4439=ORIENTED_EDGE('',*,*,#3518,.F.);
#4440=ORIENTED_EDGE('',*,*,#3519,.T.);
#4441=ORIENTED_EDGE('',*,*,#3505,.T.);
#4442=ORIENTED_EDGE('',*,*,#3519,.F.);
#4443=ORIENTED_EDGE('',*,*,#3520,.F.);
#4444=ORIENTED_EDGE('',*,*,#3521,.T.);
#4445=ORIENTED_EDGE('',*,*,#3509,.T.);
#4446=ORIENTED_EDGE('',*,*,#3521,.F.);
#4447=ORIENTED_EDGE('',*,*,#3522,.F.);
#4448=ORIENTED_EDGE('',*,*,#3523,.T.);
#4449=ORIENTED_EDGE('',*,*,#3513,.T.);
#4450=ORIENTED_EDGE('',*,*,#3523,.F.);
#4451=ORIENTED_EDGE('',*,*,#3524,.F.);
#4452=ORIENTED_EDGE('',*,*,#3525,.T.);
#4453=ORIENTED_EDGE('',*,*,#3517,.T.);
#4454=ORIENTED_EDGE('',*,*,#3525,.F.);
#4455=ORIENTED_EDGE('',*,*,#3526,.T.);
#4456=ORIENTED_EDGE('',*,*,#3527,.T.);
#4457=ORIENTED_EDGE('',*,*,#3528,.F.);
#4458=ORIENTED_EDGE('',*,*,#3529,.F.);
#4459=ORIENTED_EDGE('',*,*,#3530,.T.);
#4460=ORIENTED_EDGE('',*,*,#3529,.T.);
#4461=ORIENTED_EDGE('',*,*,#3531,.F.);
#4462=ORIENTED_EDGE('',*,*,#3532,.F.);
#4463=ORIENTED_EDGE('',*,*,#3501,.T.);
#4464=ORIENTED_EDGE('',*,*,#3533,.T.);
#4465=ORIENTED_EDGE('',*,*,#3532,.T.);
#4466=ORIENTED_EDGE('',*,*,#3534,.F.);
#4467=ORIENTED_EDGE('',*,*,#3535,.F.);
#4468=ORIENTED_EDGE('',*,*,#3446,.T.);
#4469=ORIENTED_EDGE('',*,*,#3461,.T.);
#4470=ORIENTED_EDGE('',*,*,#3476,.T.);
#4471=ORIENTED_EDGE('',*,*,#3491,.T.);
#4472=ORIENTED_EDGE('',*,*,#3536,.T.);
#4473=ORIENTED_EDGE('',*,*,#3535,.T.);
#4474=ORIENTED_EDGE('',*,*,#3537,.F.);
#4475=ORIENTED_EDGE('',*,*,#3527,.F.);
#4476=ORIENTED_EDGE('',*,*,#3494,.T.);
#4477=ORIENTED_EDGE('',*,*,#3537,.T.);
#4478=ORIENTED_EDGE('',*,*,#3534,.T.);
#4479=ORIENTED_EDGE('',*,*,#3531,.T.);
#4480=ORIENTED_EDGE('',*,*,#3528,.T.);
#4481=ORIENTED_EDGE('',*,*,#3441,.T.);
#4482=ORIENTED_EDGE('',*,*,#3456,.T.);
#4483=ORIENTED_EDGE('',*,*,#3471,.T.);
#4484=ORIENTED_EDGE('',*,*,#3486,.T.);
#4485=ORIENTED_EDGE('',*,*,#3516,.T.);
#4486=ORIENTED_EDGE('',*,*,#3512,.T.);
#4487=ORIENTED_EDGE('',*,*,#3508,.T.);
#4488=ORIENTED_EDGE('',*,*,#3504,.T.);
#4489=ORIENTED_EDGE('',*,*,#3433,.T.);
#4490=ORIENTED_EDGE('',*,*,#3536,.F.);
#4491=ORIENTED_EDGE('',*,*,#3526,.F.);
#4492=ORIENTED_EDGE('',*,*,#3530,.F.);
#4493=ORIENTED_EDGE('',*,*,#3533,.F.);
#4494=ORIENTED_EDGE('',*,*,#3518,.T.);
#4495=ORIENTED_EDGE('',*,*,#3520,.T.);
#4496=ORIENTED_EDGE('',*,*,#3522,.T.);
#4497=ORIENTED_EDGE('',*,*,#3524,.T.);
#5572=CYLINDRICAL_SURFACE('',#6579,0.4);
#5573=CYLINDRICAL_SURFACE('',#6584,0.4);
#5574=CYLINDRICAL_SURFACE('',#6587,0.4);
#5575=CYLINDRICAL_SURFACE('',#6597,0.4);
#5576=CYLINDRICAL_SURFACE('',#6598,0.4);
#5577=CYLINDRICAL_SURFACE('',#6600,0.4);
#5578=CYLINDRICAL_SURFACE('',#6603,0.685);
#5579=CYLINDRICAL_SURFACE('',#6607,0.15);
#5580=CYLINDRICAL_SURFACE('',#6609,0.25);
#5581=CYLINDRICAL_SURFACE('',#6613,0.2);
#5582=CYLINDRICAL_SURFACE('',#6615,0.515);
#5583=CYLINDRICAL_SURFACE('',#6619,0.15);
#5584=CYLINDRICAL_SURFACE('',#6621,0.25);
#5585=CYLINDRICAL_SURFACE('',#6625,0.2);
#5586=CYLINDRICAL_SURFACE('',#6627,0.515);
#5587=CYLINDRICAL_SURFACE('',#6631,0.15);
#5588=CYLINDRICAL_SURFACE('',#6633,0.25);
#5589=CYLINDRICAL_SURFACE('',#6637,0.2);
#5590=CYLINDRICAL_SURFACE('',#6639,0.515);
#5591=CYLINDRICAL_SURFACE('',#6643,0.15);
#5592=CYLINDRICAL_SURFACE('',#6645,0.25);
#5593=CYLINDRICAL_SURFACE('',#6649,0.2);
#5594=CYLINDRICAL_SURFACE('',#6651,0.515);
#5595=CYLINDRICAL_SURFACE('',#6655,0.3);
#5596=CYLINDRICAL_SURFACE('',#6658,0.4);
#5597=CYLINDRICAL_SURFACE('',#6663,0.4);
#5598=CYLINDRICAL_SURFACE('',#6668,0.4);
#5599=CYLINDRICAL_SURFACE('',#6673,0.4);
#5600=CYLINDRICAL_SURFACE('',#6678,0.225);
#5601=CYLINDRICAL_SURFACE('',#6680,0.225);
#5602=CYLINDRICAL_SURFACE('',#6682,0.225);
#5603=CYLINDRICAL_SURFACE('',#6684,0.225);
#5733=ADVANCED_FACE('',(#834),#594,.T.);
#5734=ADVANCED_FACE('',(#835),#595,.T.);
#5735=ADVANCED_FACE('',(#836),#596,.F.);
#5736=ADVANCED_FACE('',(#837),#5572,.F.);
#5737=ADVANCED_FACE('',(#838),#5573,.F.);
#5738=ADVANCED_FACE('',(#839),#5574,.F.);
#5739=ADVANCED_FACE('',(#840),#597,.F.);
#5740=ADVANCED_FACE('',(#841),#598,.T.);
#5741=ADVANCED_FACE('',(#842),#599,.T.);
#5742=ADVANCED_FACE('',(#843),#600,.T.);
#5743=ADVANCED_FACE('',(#844),#5575,.F.);
#5744=ADVANCED_FACE('',(#845),#5576,.F.);
#5745=ADVANCED_FACE('',(#846),#5577,.F.);
#5746=ADVANCED_FACE('',(#847),#601,.T.);
#5747=ADVANCED_FACE('',(#848),#5578,.F.);
#5748=ADVANCED_FACE('',(#849,#424),#602,.T.);
#5749=ADVANCED_FACE('',(#850),#5579,.F.);
#5750=ADVANCED_FACE('',(#851),#5580,.F.);
#5751=ADVANCED_FACE('',(#852,#425),#603,.T.);
#5752=ADVANCED_FACE('',(#853),#5581,.F.);
#5753=ADVANCED_FACE('',(#854),#5582,.F.);
#5754=ADVANCED_FACE('',(#855,#426),#604,.F.);
#5755=ADVANCED_FACE('',(#856),#5583,.F.);
#5756=ADVANCED_FACE('',(#857),#5584,.F.);
#5757=ADVANCED_FACE('',(#858,#427),#605,.T.);
#5758=ADVANCED_FACE('',(#859),#5585,.F.);
#5759=ADVANCED_FACE('',(#860),#5586,.F.);
#5760=ADVANCED_FACE('',(#861,#428),#606,.F.);
#5761=ADVANCED_FACE('',(#862),#5587,.F.);
#5762=ADVANCED_FACE('',(#863),#5588,.F.);
#5763=ADVANCED_FACE('',(#864,#429),#607,.T.);
#5764=ADVANCED_FACE('',(#865),#5589,.F.);
#5765=ADVANCED_FACE('',(#866),#5590,.F.);
#5766=ADVANCED_FACE('',(#867,#430),#608,.F.);
#5767=ADVANCED_FACE('',(#868),#5591,.F.);
#5768=ADVANCED_FACE('',(#869),#5592,.F.);
#5769=ADVANCED_FACE('',(#870,#431),#609,.T.);
#5770=ADVANCED_FACE('',(#871),#5593,.F.);
#5771=ADVANCED_FACE('',(#872),#5594,.F.);
#5772=ADVANCED_FACE('',(#873,#432),#610,.F.);
#5773=ADVANCED_FACE('',(#874,#433,#434,#435,#436),#5595,.F.);
#5774=ADVANCED_FACE('',(#875),#5596,.F.);
#5775=ADVANCED_FACE('',(#876,#437),#611,.T.);
#5776=ADVANCED_FACE('',(#877),#5597,.F.);
#5777=ADVANCED_FACE('',(#878,#438),#612,.T.);
#5778=ADVANCED_FACE('',(#879),#5598,.F.);
#5779=ADVANCED_FACE('',(#880,#439),#613,.T.);
#5780=ADVANCED_FACE('',(#881),#5599,.F.);
#5781=ADVANCED_FACE('',(#882,#440),#614,.T.);
#5782=ADVANCED_FACE('',(#883),#5600,.F.);
#5783=ADVANCED_FACE('',(#884),#5601,.F.);
#5784=ADVANCED_FACE('',(#885),#5602,.F.);
#5785=ADVANCED_FACE('',(#886),#5603,.F.);
#5786=ADVANCED_FACE('',(#887),#615,.T.);
#5787=ADVANCED_FACE('',(#888,#441),#616,.T.);
#5788=ADVANCED_FACE('',(#889,#442,#443,#444,#445),#617,.T.);
#5789=ADVANCED_FACE('',(#890,#446),#618,.T.);
#5790=ADVANCED_FACE('',(#891,#447,#448,#449,#450,#451,#452,#453,#454,#455),
#619,.T.);
#5791=ADVANCED_FACE('',(#892,#456,#457,#458,#459),#620,.F.);
#6070=CLOSED_SHELL('',(#5733,#5734,#5735,#5736,#5737,#5738,#5739,#5740,
#5741,#5742,#5743,#5744,#5745,#5746,#5747,#5748,#5749,#5750,#5751,#5752,
#5753,#5754,#5755,#5756,#5757,#5758,#5759,#5760,#5761,#5762,#5763,#5764,
#5765,#5766,#5767,#5768,#5769,#5770,#5771,#5772,#5773,#5774,#5775,#5776,
#5777,#5778,#5779,#5780,#5781,#5782,#5783,#5784,#5785,#5786,#5787,#5788,
#5789,#5790,#5791));
#6572=AXIS2_PLACEMENT_3D('',#9364,#7449,#7450);
#6573=AXIS2_PLACEMENT_3D('',#9365,#7451,#7452);
#6574=AXIS2_PLACEMENT_3D('',#9369,#7454,#7455);
#6575=AXIS2_PLACEMENT_3D('',#9370,#7456,#7457);
#6576=AXIS2_PLACEMENT_3D('',#9373,#7459,#7460);
#6577=AXIS2_PLACEMENT_3D('',#9374,#7461,#7462);
#6578=AXIS2_PLACEMENT_3D('',#9378,#7464,#7465);
#6579=AXIS2_PLACEMENT_3D('',#9379,#7466,#7467);
#6580=AXIS2_PLACEMENT_3D('',#9385,#7470,#7471);
#6581=AXIS2_PLACEMENT_3D('',#9387,#7472,#7473);
#6582=AXIS2_PLACEMENT_3D('',#9445,#7475,#7476);
#6583=AXIS2_PLACEMENT_3D('',#9463,#7477,#7478);
#6584=AXIS2_PLACEMENT_3D('',#9464,#7479,#7480);
#6585=AXIS2_PLACEMENT_3D('',#9465,#7481,#7482);
#6586=AXIS2_PLACEMENT_3D('',#9466,#7483,#7484);
#6587=AXIS2_PLACEMENT_3D('',#9467,#7485,#7486);
#6588=AXIS2_PLACEMENT_3D('',#9469,#7487,#7488);
#6589=AXIS2_PLACEMENT_3D('',#9470,#7489,#7490);
#6590=AXIS2_PLACEMENT_3D('',#9471,#7491,#7492);
#6591=AXIS2_PLACEMENT_3D('',#9472,#7493,#7494);
#6592=AXIS2_PLACEMENT_3D('',#9474,#7496,#7497);
#6593=AXIS2_PLACEMENT_3D('',#9476,#7499,#7500);
#6594=AXIS2_PLACEMENT_3D('',#9477,#7501,#7502);
#6595=AXIS2_PLACEMENT_3D('',#9478,#7503,#7504);
#6596=AXIS2_PLACEMENT_3D('',#9479,#7505,#7506);
#6597=AXIS2_PLACEMENT_3D('',#9480,#7507,#7508);
#6598=AXIS2_PLACEMENT_3D('',#9481,#7509,#7510);
#6599=AXIS2_PLACEMENT_3D('',#9484,#7512,#7513);
#6600=AXIS2_PLACEMENT_3D('',#9485,#7514,#7515);
#6601=AXIS2_PLACEMENT_3D('',#9486,#7516,#7517);
#6602=AXIS2_PLACEMENT_3D('',#9487,#7518,#7519);
#6603=AXIS2_PLACEMENT_3D('',#9488,#7520,#7521);
#6604=AXIS2_PLACEMENT_3D('',#9490,#7522,#7523);
#6605=AXIS2_PLACEMENT_3D('',#9493,#7525,#7526);
#6606=AXIS2_PLACEMENT_3D('',#9494,#7527,#7528);
#6607=AXIS2_PLACEMENT_3D('',#9495,#7529,#7530);
#6608=AXIS2_PLACEMENT_3D('',#9521,#7532,#7533);
#6609=AXIS2_PLACEMENT_3D('',#9540,#7534,#7535);
#6610=AXIS2_PLACEMENT_3D('',#9542,#7536,#7537);
#6611=AXIS2_PLACEMENT_3D('',#9545,#7539,#7540);
#6612=AXIS2_PLACEMENT_3D('',#9546,#7541,#7542);
#6613=AXIS2_PLACEMENT_3D('',#9547,#7543,#7544);
#6614=AXIS2_PLACEMENT_3D('',#9549,#7545,#7546);
#6615=AXIS2_PLACEMENT_3D('',#9589,#7548,#7549);
#6616=AXIS2_PLACEMENT_3D('',#9591,#7550,#7551);
#6617=AXIS2_PLACEMENT_3D('',#9594,#7553,#7554);
#6618=AXIS2_PLACEMENT_3D('',#9595,#7555,#7556);
#6619=AXIS2_PLACEMENT_3D('',#9596,#7557,#7558);
#6620=AXIS2_PLACEMENT_3D('',#9622,#7560,#7561);
#6621=AXIS2_PLACEMENT_3D('',#9641,#7562,#7563);
#6622=AXIS2_PLACEMENT_3D('',#9643,#7564,#7565);
#6623=AXIS2_PLACEMENT_3D('',#9646,#7567,#7568);
#6624=AXIS2_PLACEMENT_3D('',#9647,#7569,#7570);
#6625=AXIS2_PLACEMENT_3D('',#9648,#7571,#7572);
#6626=AXIS2_PLACEMENT_3D('',#9650,#7573,#7574);
#6627=AXIS2_PLACEMENT_3D('',#9690,#7576,#7577);
#6628=AXIS2_PLACEMENT_3D('',#9692,#7578,#7579);
#6629=AXIS2_PLACEMENT_3D('',#9695,#7581,#7582);
#6630=AXIS2_PLACEMENT_3D('',#9696,#7583,#7584);
#6631=AXIS2_PLACEMENT_3D('',#9697,#7585,#7586);
#6632=AXIS2_PLACEMENT_3D('',#9723,#7588,#7589);
#6633=AXIS2_PLACEMENT_3D('',#9742,#7590,#7591);
#6634=AXIS2_PLACEMENT_3D('',#9744,#7592,#7593);
#6635=AXIS2_PLACEMENT_3D('',#9747,#7595,#7596);
#6636=AXIS2_PLACEMENT_3D('',#9748,#7597,#7598);
#6637=AXIS2_PLACEMENT_3D('',#9749,#7599,#7600);
#6638=AXIS2_PLACEMENT_3D('',#9751,#7601,#7602);
#6639=AXIS2_PLACEMENT_3D('',#9791,#7604,#7605);
#6640=AXIS2_PLACEMENT_3D('',#9793,#7606,#7607);
#6641=AXIS2_PLACEMENT_3D('',#9796,#7609,#7610);
#6642=AXIS2_PLACEMENT_3D('',#9797,#7611,#7612);
#6643=AXIS2_PLACEMENT_3D('',#9798,#7613,#7614);
#6644=AXIS2_PLACEMENT_3D('',#9824,#7616,#7617);
#6645=AXIS2_PLACEMENT_3D('',#9843,#7618,#7619);
#6646=AXIS2_PLACEMENT_3D('',#9845,#7620,#7621);
#6647=AXIS2_PLACEMENT_3D('',#9848,#7623,#7624);
#6648=AXIS2_PLACEMENT_3D('',#9849,#7625,#7626);
#6649=AXIS2_PLACEMENT_3D('',#9850,#7627,#7628);
#6650=AXIS2_PLACEMENT_3D('',#9852,#7629,#7630);
#6651=AXIS2_PLACEMENT_3D('',#9892,#7632,#7633);
#6652=AXIS2_PLACEMENT_3D('',#9894,#7634,#7635);
#6653=AXIS2_PLACEMENT_3D('',#9897,#7637,#7638);
#6654=AXIS2_PLACEMENT_3D('',#9898,#7639,#7640);
#6655=AXIS2_PLACEMENT_3D('',#9899,#7641,#7642);
#6656=AXIS2_PLACEMENT_3D('',#9901,#7643,#7644);
#6657=AXIS2_PLACEMENT_3D('',#9909,#7651,#7652);
#6658=AXIS2_PLACEMENT_3D('',#9910,#7653,#7654);
#6659=AXIS2_PLACEMENT_3D('',#9912,#7655,#7656);
#6660=AXIS2_PLACEMENT_3D('',#9915,#7658,#7659);
#6661=AXIS2_PLACEMENT_3D('',#9916,#7660,#7661);
#6662=AXIS2_PLACEMENT_3D('',#9918,#7662,#7663);
#6663=AXIS2_PLACEMENT_3D('',#9919,#7664,#7665);
#6664=AXIS2_PLACEMENT_3D('',#9921,#7666,#7667);
#6665=AXIS2_PLACEMENT_3D('',#9924,#7669,#7670);
#6666=AXIS2_PLACEMENT_3D('',#9925,#7671,#7672);
#6667=AXIS2_PLACEMENT_3D('',#9927,#7673,#7674);
#6668=AXIS2_PLACEMENT_3D('',#9928,#7675,#7676);
#6669=AXIS2_PLACEMENT_3D('',#9930,#7677,#7678);
#6670=AXIS2_PLACEMENT_3D('',#9933,#7680,#7681);
#6671=AXIS2_PLACEMENT_3D('',#9934,#7682,#7683);
#6672=AXIS2_PLACEMENT_3D('',#9936,#7684,#7685);
#6673=AXIS2_PLACEMENT_3D('',#9937,#7686,#7687);
#6674=AXIS2_PLACEMENT_3D('',#9939,#7688,#7689);
#6675=AXIS2_PLACEMENT_3D('',#9942,#7691,#7692);
#6676=AXIS2_PLACEMENT_3D('',#9943,#7693,#7694);
#6677=AXIS2_PLACEMENT_3D('',#9945,#7695,#7696);
#6678=AXIS2_PLACEMENT_3D('',#9946,#7697,#7698);
#6679=AXIS2_PLACEMENT_3D('',#9948,#7699,#7700);
#6680=AXIS2_PLACEMENT_3D('',#9950,#7702,#7703);
#6681=AXIS2_PLACEMENT_3D('',#9952,#7704,#7705);
#6682=AXIS2_PLACEMENT_3D('',#9954,#7707,#7708);
#6683=AXIS2_PLACEMENT_3D('',#9956,#7709,#7710);
#6684=AXIS2_PLACEMENT_3D('',#9958,#7712,#7713);
#6685=AXIS2_PLACEMENT_3D('',#9960,#7714,#7715);
#6686=AXIS2_PLACEMENT_3D('',#9962,#7717,#7718);
#6687=AXIS2_PLACEMENT_3D('',#9971,#7723,#7724);
#6688=AXIS2_PLACEMENT_3D('',#9977,#7728,#7729);
#6689=AXIS2_PLACEMENT_3D('',#9983,#7733,#7734);
#6690=AXIS2_PLACEMENT_3D('',#9986,#7737,#7738);
#6691=AXIS2_PLACEMENT_3D('',#9987,#7739,#7740);
#7449=DIRECTION('axis',(0.,0.,1.));
#7450=DIRECTION('refdir',(1.,0.,0.));
#7451=DIRECTION('center_axis',(0.,1.,0.));
#7452=DIRECTION('ref_axis',(1.,0.,0.));
#7453=DIRECTION('',(-1.,0.,0.));
#7454=DIRECTION('center_axis',(0.,1.,0.));
#7455=DIRECTION('ref_axis',(1.,0.,0.));
#7456=DIRECTION('center_axis',(0.,1.,0.));
#7457=DIRECTION('ref_axis',(1.,0.,0.));
#7458=DIRECTION('',(0.,0.,-1.));
#7459=DIRECTION('center_axis',(0.,1.,0.));
#7460=DIRECTION('ref_axis',(1.,0.,0.));
#7461=DIRECTION('center_axis',(0.,1.,0.));
#7462=DIRECTION('ref_axis',(1.,0.,0.));
#7463=DIRECTION('',(-1.,0.,0.));
#7464=DIRECTION('center_axis',(0.,1.,0.));
#7465=DIRECTION('ref_axis',(1.,0.,0.));
#7466=DIRECTION('center_axis',(0.,1.,0.));
#7467=DIRECTION('ref_axis',(1.,0.,0.));
#7468=DIRECTION('',(0.,1.,0.));
#7469=DIRECTION('',(0.,-1.,0.));
#7470=DIRECTION('center_axis',(0.,0.707106781186548,0.707106781186547));
#7471=DIRECTION('ref_axis',(0.,0.707106781186547,-0.707106781186548));
#7472=DIRECTION('center_axis',(0.,0.707106781186548,-0.707106781186547));
#7473=DIRECTION('ref_axis',(0.,-0.707106781186547,-0.707106781186548));
#7474=DIRECTION('',(0.,1.,0.));
#7475=DIRECTION('center_axis',(0.,1.,0.));
#7476=DIRECTION('ref_axis',(1.,0.,0.));
#7477=DIRECTION('center_axis',(0.,0.707106781186548,0.707106781186547));
#7478=DIRECTION('ref_axis',(0.,0.707106781186547,-0.707106781186548));
#7479=DIRECTION('center_axis',(0.,1.,0.));
#7480=DIRECTION('ref_axis',(1.,0.,0.));
#7481=DIRECTION('center_axis',(0.,-0.707106781186548,-0.707106781186547));
#7482=DIRECTION('ref_axis',(0.,0.707106781186547,-0.707106781186548));
#7483=DIRECTION('center_axis',(0.,-0.707106781186548,0.707106781186547));
#7484=DIRECTION('ref_axis',(0.,-0.707106781186547,-0.707106781186548));
#7485=DIRECTION('center_axis',(0.,1.,0.));
#7486=DIRECTION('ref_axis',(-1.,0.,1.22464679914735E-16));
#7487=DIRECTION('center_axis',(0.,-0.707106781186548,-0.707106781186547));
#7488=DIRECTION('ref_axis',(0.,0.707106781186547,-0.707106781186548));
#7489=DIRECTION('center_axis',(0.,1.,0.));
#7490=DIRECTION('ref_axis',(1.,0.,0.));
#7491=DIRECTION('center_axis',(0.,-0.707106781186548,0.707106781186547));
#7492=DIRECTION('ref_axis',(0.,-0.707106781186547,-0.707106781186548));
#7493=DIRECTION('center_axis',(0.,1.,0.));
#7494=DIRECTION('ref_axis',(1.,0.,0.));
#7495=DIRECTION('',(1.,0.,0.));
#7496=DIRECTION('center_axis',(0.,1.,0.));
#7497=DIRECTION('ref_axis',(1.,0.,0.));
#7498=DIRECTION('',(0.,0.,1.));
#7499=DIRECTION('center_axis',(0.,0.,1.));
#7500=DIRECTION('ref_axis',(1.,0.,0.));
#7501=DIRECTION('center_axis',(0.,0.,1.));
#7502=DIRECTION('ref_axis',(1.,0.,0.));
#7503=DIRECTION('center_axis',(0.,0.,1.));
#7504=DIRECTION('ref_axis',(1.,0.,0.));
#7505=DIRECTION('center_axis',(0.,0.,1.));
#7506=DIRECTION('ref_axis',(1.,0.,0.));
#7507=DIRECTION('center_axis',(0.,0.,1.));
#7508=DIRECTION('ref_axis',(1.,0.,0.));
#7509=DIRECTION('center_axis',(0.,0.,1.));
#7510=DIRECTION('ref_axis',(1.,0.,0.));
#7511=DIRECTION('',(0.,0.,1.));
#7512=DIRECTION('center_axis',(0.,0.,-1.));
#7513=DIRECTION('ref_axis',(1.,0.,0.));
#7514=DIRECTION('center_axis',(0.,0.,1.));
#7515=DIRECTION('ref_axis',(-1.,1.22464679914735E-16,0.));
#7516=DIRECTION('center_axis',(0.,0.,1.));
#7517=DIRECTION('ref_axis',(1.,0.,0.));
#7518=DIRECTION('center_axis',(0.,0.,1.));
#7519=DIRECTION('ref_axis',(1.,0.,0.));
#7520=DIRECTION('center_axis',(0.,0.,1.));
#7521=DIRECTION('ref_axis',(1.,0.,0.));
#7522=DIRECTION('center_axis',(0.,0.,1.));
#7523=DIRECTION('ref_axis',(1.,0.,0.));
#7524=DIRECTION('',(0.,0.,1.));
#7525=DIRECTION('center_axis',(0.,0.,-1.));
#7526=DIRECTION('ref_axis',(1.,0.,0.));
#7527=DIRECTION('center_axis',(0.,0.,1.));
#7528=DIRECTION('ref_axis',(1.,0.,0.));
#7529=DIRECTION('center_axis',(0.,0.,1.));
#7530=DIRECTION('ref_axis',(1.,0.,0.));
#7531=DIRECTION('',(0.,0.,1.));
#7532=DIRECTION('center_axis',(0.,0.,-1.));
#7533=DIRECTION('ref_axis',(1.,0.,0.));
#7534=DIRECTION('center_axis',(0.,0.,1.));
#7535=DIRECTION('ref_axis',(1.,0.,0.));
#7536=DIRECTION('center_axis',(0.,0.,1.));
#7537=DIRECTION('ref_axis',(1.,0.,0.));
#7538=DIRECTION('',(0.,0.,1.));
#7539=DIRECTION('center_axis',(0.,0.,-1.));
#7540=DIRECTION('ref_axis',(1.,0.,0.));
#7541=DIRECTION('center_axis',(0.,0.,1.));
#7542=DIRECTION('ref_axis',(1.,0.,0.));
#7543=DIRECTION('center_axis',(0.,1.,0.));
#7544=DIRECTION('ref_axis',(1.,0.,0.));
#7545=DIRECTION('center_axis',(0.,1.,0.));
#7546=DIRECTION('ref_axis',(1.,0.,0.));
#7547=DIRECTION('',(0.,1.,0.));
#7548=DIRECTION('center_axis',(0.,1.,0.));
#7549=DIRECTION('ref_axis',(1.,0.,0.));
#7550=DIRECTION('center_axis',(0.,1.,0.));
#7551=DIRECTION('ref_axis',(1.,0.,0.));
#7552=DIRECTION('',(0.,1.,0.));
#7553=DIRECTION('center_axis',(0.,1.,0.));
#7554=DIRECTION('ref_axis',(1.,0.,0.));
#7555=DIRECTION('center_axis',(0.,1.,0.));
#7556=DIRECTION('ref_axis',(1.,0.,0.));
#7557=DIRECTION('center_axis',(0.,0.,1.));
#7558=DIRECTION('ref_axis',(1.,0.,0.));
#7559=DIRECTION('',(0.,0.,1.));
#7560=DIRECTION('center_axis',(0.,0.,-1.));
#7561=DIRECTION('ref_axis',(1.,0.,0.));
#7562=DIRECTION('center_axis',(0.,0.,1.));
#7563=DIRECTION('ref_axis',(1.,0.,0.));
#7564=DIRECTION('center_axis',(0.,0.,1.));
#7565=DIRECTION('ref_axis',(1.,0.,0.));
#7566=DIRECTION('',(0.,0.,1.));
#7567=DIRECTION('center_axis',(0.,0.,-1.));
#7568=DIRECTION('ref_axis',(1.,0.,0.));
#7569=DIRECTION('center_axis',(0.,0.,1.));
#7570=DIRECTION('ref_axis',(1.,0.,0.));
#7571=DIRECTION('center_axis',(0.,1.,0.));
#7572=DIRECTION('ref_axis',(1.,0.,0.));
#7573=DIRECTION('center_axis',(0.,1.,0.));
#7574=DIRECTION('ref_axis',(1.,0.,0.));
#7575=DIRECTION('',(0.,1.,0.));
#7576=DIRECTION('center_axis',(0.,1.,0.));
#7577=DIRECTION('ref_axis',(1.,0.,0.));
#7578=DIRECTION('center_axis',(0.,1.,0.));
#7579=DIRECTION('ref_axis',(1.,0.,0.));
#7580=DIRECTION('',(0.,1.,0.));
#7581=DIRECTION('center_axis',(0.,1.,0.));
#7582=DIRECTION('ref_axis',(1.,0.,0.));
#7583=DIRECTION('center_axis',(0.,1.,0.));
#7584=DIRECTION('ref_axis',(1.,0.,0.));
#7585=DIRECTION('center_axis',(0.,0.,1.));
#7586=DIRECTION('ref_axis',(1.,0.,0.));
#7587=DIRECTION('',(0.,0.,1.));
#7588=DIRECTION('center_axis',(0.,0.,-1.));
#7589=DIRECTION('ref_axis',(1.,0.,0.));
#7590=DIRECTION('center_axis',(0.,0.,1.));
#7591=DIRECTION('ref_axis',(1.,0.,0.));
#7592=DIRECTION('center_axis',(0.,0.,1.));
#7593=DIRECTION('ref_axis',(1.,0.,0.));
#7594=DIRECTION('',(0.,0.,1.));
#7595=DIRECTION('center_axis',(0.,0.,-1.));
#7596=DIRECTION('ref_axis',(1.,0.,0.));
#7597=DIRECTION('center_axis',(0.,0.,1.));
#7598=DIRECTION('ref_axis',(1.,0.,0.));
#7599=DIRECTION('center_axis',(0.,1.,0.));
#7600=DIRECTION('ref_axis',(1.,0.,0.));
#7601=DIRECTION('center_axis',(0.,1.,0.));
#7602=DIRECTION('ref_axis',(1.,0.,0.));
#7603=DIRECTION('',(0.,1.,0.));
#7604=DIRECTION('center_axis',(0.,1.,0.));
#7605=DIRECTION('ref_axis',(1.,0.,0.));
#7606=DIRECTION('center_axis',(0.,1.,0.));
#7607=DIRECTION('ref_axis',(1.,0.,0.));
#7608=DIRECTION('',(0.,1.,0.));
#7609=DIRECTION('center_axis',(0.,1.,0.));
#7610=DIRECTION('ref_axis',(1.,0.,0.));
#7611=DIRECTION('center_axis',(0.,1.,0.));
#7612=DIRECTION('ref_axis',(1.,0.,0.));
#7613=DIRECTION('center_axis',(0.,0.,1.));
#7614=DIRECTION('ref_axis',(1.,0.,0.));
#7615=DIRECTION('',(0.,0.,1.));
#7616=DIRECTION('center_axis',(0.,0.,-1.));
#7617=DIRECTION('ref_axis',(1.,0.,0.));
#7618=DIRECTION('center_axis',(0.,0.,1.));
#7619=DIRECTION('ref_axis',(1.,0.,0.));
#7620=DIRECTION('center_axis',(0.,0.,1.));
#7621=DIRECTION('ref_axis',(1.,0.,0.));
#7622=DIRECTION('',(0.,0.,1.));
#7623=DIRECTION('center_axis',(0.,0.,-1.));
#7624=DIRECTION('ref_axis',(1.,0.,0.));
#7625=DIRECTION('center_axis',(0.,0.,1.));
#7626=DIRECTION('ref_axis',(1.,0.,0.));
#7627=DIRECTION('center_axis',(0.,1.,0.));
#7628=DIRECTION('ref_axis',(1.,0.,0.));
#7629=DIRECTION('center_axis',(0.,1.,0.));
#7630=DIRECTION('ref_axis',(1.,0.,0.));
#7631=DIRECTION('',(0.,1.,0.));
#7632=DIRECTION('center_axis',(0.,1.,0.));
#7633=DIRECTION('ref_axis',(1.,0.,0.));
#7634=DIRECTION('center_axis',(0.,1.,0.));
#7635=DIRECTION('ref_axis',(1.,0.,0.));
#7636=DIRECTION('',(0.,1.,0.));
#7637=DIRECTION('center_axis',(0.,1.,0.));
#7638=DIRECTION('ref_axis',(1.,0.,0.));
#7639=DIRECTION('center_axis',(0.,1.,0.));
#7640=DIRECTION('ref_axis',(1.,0.,0.));
#7641=DIRECTION('center_axis',(1.,0.,0.));
#7642=DIRECTION('ref_axis',(0.,0.,-1.));
#7643=DIRECTION('center_axis',(1.,0.,0.));
#7644=DIRECTION('ref_axis',(0.,0.,-1.));
#7645=DIRECTION('',(1.,0.,0.));
#7646=DIRECTION('',(1.,0.,0.));
#7647=DIRECTION('',(1.,0.,0.));
#7648=DIRECTION('',(1.,0.,0.));
#7649=DIRECTION('',(1.,0.,0.));
#7650=DIRECTION('',(1.,0.,0.));
#7651=DIRECTION('center_axis',(-1.,0.,0.));
#7652=DIRECTION('ref_axis',(0.,0.,-1.));
#7653=DIRECTION('center_axis',(0.,0.,1.));
#7654=DIRECTION('ref_axis',(1.,0.,0.));
#7655=DIRECTION('center_axis',(0.,0.,1.));
#7656=DIRECTION('ref_axis',(1.,0.,0.));
#7657=DIRECTION('',(0.,0.,1.));
#7658=DIRECTION('center_axis',(0.,0.,-1.));
#7659=DIRECTION('ref_axis',(1.,0.,0.));
#7660=DIRECTION('center_axis',(0.,0.,1.));
#7661=DIRECTION('ref_axis',(1.,0.,0.));
#7662=DIRECTION('center_axis',(0.,0.,1.));
#7663=DIRECTION('ref_axis',(1.,0.,0.));
#7664=DIRECTION('center_axis',(0.,0.,1.));
#7665=DIRECTION('ref_axis',(1.,0.,0.));
#7666=DIRECTION('center_axis',(0.,0.,1.));
#7667=DIRECTION('ref_axis',(1.,0.,0.));
#7668=DIRECTION('',(0.,0.,1.));
#7669=DIRECTION('center_axis',(0.,0.,-1.));
#7670=DIRECTION('ref_axis',(1.,0.,0.));
#7671=DIRECTION('center_axis',(0.,0.,1.));
#7672=DIRECTION('ref_axis',(1.,0.,0.));
#7673=DIRECTION('center_axis',(0.,0.,1.));
#7674=DIRECTION('ref_axis',(1.,0.,0.));
#7675=DIRECTION('center_axis',(0.,0.,1.));
#7676=DIRECTION('ref_axis',(1.,0.,0.));
#7677=DIRECTION('center_axis',(0.,0.,1.));
#7678=DIRECTION('ref_axis',(1.,0.,0.));
#7679=DIRECTION('',(0.,0.,1.));
#7680=DIRECTION('center_axis',(0.,0.,-1.));
#7681=DIRECTION('ref_axis',(1.,0.,0.));
#7682=DIRECTION('center_axis',(0.,0.,1.));
#7683=DIRECTION('ref_axis',(1.,0.,0.));
#7684=DIRECTION('center_axis',(0.,0.,1.));
#7685=DIRECTION('ref_axis',(1.,0.,0.));
#7686=DIRECTION('center_axis',(0.,0.,1.));
#7687=DIRECTION('ref_axis',(1.,0.,0.));
#7688=DIRECTION('center_axis',(0.,0.,1.));
#7689=DIRECTION('ref_axis',(1.,0.,0.));
#7690=DIRECTION('',(0.,0.,1.));
#7691=DIRECTION('center_axis',(0.,0.,-1.));
#7692=DIRECTION('ref_axis',(1.,0.,0.));
#7693=DIRECTION('center_axis',(0.,0.,1.));
#7694=DIRECTION('ref_axis',(1.,0.,0.));
#7695=DIRECTION('center_axis',(0.,0.,1.));
#7696=DIRECTION('ref_axis',(1.,0.,0.));
#7697=DIRECTION('center_axis',(0.,0.,1.));
#7698=DIRECTION('ref_axis',(1.,0.,0.));
#7699=DIRECTION('center_axis',(0.,0.,1.));
#7700=DIRECTION('ref_axis',(1.,0.,0.));
#7701=DIRECTION('',(0.,0.,1.));
#7702=DIRECTION('center_axis',(0.,0.,1.));
#7703=DIRECTION('ref_axis',(1.,0.,0.));
#7704=DIRECTION('center_axis',(0.,0.,1.));
#7705=DIRECTION('ref_axis',(1.,0.,0.));
#7706=DIRECTION('',(0.,0.,1.));
#7707=DIRECTION('center_axis',(0.,0.,1.));
#7708=DIRECTION('ref_axis',(1.,0.,0.));
#7709=DIRECTION('center_axis',(0.,0.,1.));
#7710=DIRECTION('ref_axis',(1.,0.,0.));
#7711=DIRECTION('',(0.,0.,1.));
#7712=DIRECTION('center_axis',(0.,0.,1.));
#7713=DIRECTION('ref_axis',(1.,0.,0.));
#7714=DIRECTION('center_axis',(0.,0.,1.));
#7715=DIRECTION('ref_axis',(1.,0.,0.));
#7716=DIRECTION('',(0.,0.,1.));
#7717=DIRECTION('center_axis',(0.,1.,0.));
#7718=DIRECTION('ref_axis',(-1.,0.,0.));
#7719=DIRECTION('',(-1.,0.,0.));
#7720=DIRECTION('',(0.,0.,1.));
#7721=DIRECTION('',(-1.,0.,0.));
#7722=DIRECTION('',(0.,0.,1.));
#7723=DIRECTION('center_axis',(1.,0.,0.));
#7724=DIRECTION('ref_axis',(0.,1.,0.));
#7725=DIRECTION('',(0.,1.,0.));
#7726=DIRECTION('',(0.,1.,0.));
#7727=DIRECTION('',(0.,0.,1.));
#7728=DIRECTION('center_axis',(0.,-1.,0.));
#7729=DIRECTION('ref_axis',(1.,0.,0.));
#7730=DIRECTION('',(1.,0.,0.));
#7731=DIRECTION('',(1.,0.,0.));
#7732=DIRECTION('',(0.,0.,1.));
#7733=DIRECTION('center_axis',(-1.,0.,0.));
#7734=DIRECTION('ref_axis',(0.,-1.,0.));
#7735=DIRECTION('',(0.,-1.,0.));
#7736=DIRECTION('',(0.,-1.,0.));
#7737=DIRECTION('center_axis',(0.,0.,1.));
#7738=DIRECTION('ref_axis',(1.,0.,0.));
#7739=DIRECTION('center_axis',(0.,0.,1.));
#7740=DIRECTION('ref_axis',(1.,0.,0.));
#9364=CARTESIAN_POINT('',(0.,0.,0.));
#9365=CARTESIAN_POINT('Origin',(0.,-0.1,4.));
#9366=CARTESIAN_POINT('',(0.387298334620742,-0.1,3.9));
#9367=CARTESIAN_POINT('',(-0.387298334620742,-0.1,3.9));
#9368=CARTESIAN_POINT('',(0.,-0.1,3.9));
#9369=CARTESIAN_POINT('Origin',(0.,-0.1,4.));
#9370=CARTESIAN_POINT('Origin',(0.,-0.1,4.));
#9371=CARTESIAN_POINT('',(0.387298334620742,-0.1,4.1));
#9372=CARTESIAN_POINT('',(0.387298334620742,-0.1,3.9));
#9373=CARTESIAN_POINT('Origin',(0.,-0.1,4.));
#9374=CARTESIAN_POINT('Origin',(0.,1.6,4.));
#9375=CARTESIAN_POINT('',(0.28284271247462,1.6,4.28284271247462));
#9376=CARTESIAN_POINT('',(-0.28284271247462,1.6,4.28284271247462));
#9377=CARTESIAN_POINT('',(-5.6,1.6,4.28284271247462));
#9378=CARTESIAN_POINT('Origin',(0.,1.6,4.));
#9379=CARTESIAN_POINT('Origin',(0.,-0.1,4.));
#9380=CARTESIAN_POINT('',(-0.387298334620742,0.0999999999999997,3.9));
#9381=CARTESIAN_POINT('',(-0.387298334620742,-0.1,3.9));
#9382=CARTESIAN_POINT('',(0.387298334620742,0.0999999999999997,3.9));
#9383=CARTESIAN_POINT('',(0.387298334620742,-0.1,3.9));
#9384=CARTESIAN_POINT('',(0.4,0.,4.));
#9385=CARTESIAN_POINT('Origin',(0.,0.,4.));
#9386=CARTESIAN_POINT('',(-0.4,0.,4.));
#9387=CARTESIAN_POINT('Origin',(0.,0.,4.));
#9388=CARTESIAN_POINT('',(-0.4,1.2,4.));
#9389=CARTESIAN_POINT('',(-0.4,-0.1,4.));
#9390=CARTESIAN_POINT('',(-0.264575131106459,1.5,4.3));
#9391=CARTESIAN_POINT('Ctrl Pts',(-0.264575131106459,1.5,4.3));
#9392=CARTESIAN_POINT('Ctrl Pts',(-0.264575131106459,1.47985532278493,4.3));
#9393=CARTESIAN_POINT('Ctrl Pts',(-0.266946656583193,1.4596364158444,4.2979507721165));
#9394=CARTESIAN_POINT('Ctrl Pts',(-0.275663470560297,1.42025634008317,4.28990486485683));
#9395=CARTESIAN_POINT('Ctrl Pts',(-0.281970270384709,1.40108570205275,4.28391288325358));
#9396=CARTESIAN_POINT('Ctrl Pts',(-0.304063569802551,1.34650091982942,4.2607687447172));
#9397=CARTESIAN_POINT('Ctrl Pts',(-0.322818652826944,1.31392187404012,4.23818594275205));
#9398=CARTESIAN_POINT('Ctrl Pts',(-0.35507155223138,1.26236205014611,4.18662611885804));
#9399=CARTESIAN_POINT('Ctrl Pts',(-0.371172434841458,1.23945139911714,4.15398235555279));
#9400=CARTESIAN_POINT('Ctrl Pts',(-0.393713960479867,1.20823419970573,4.08042925305982));
#9401=CARTESIAN_POINT('Ctrl Pts',(-0.4,1.2,4.03944194682574));
#9402=CARTESIAN_POINT('Ctrl Pts',(-0.4,1.2,4.));
#9403=CARTESIAN_POINT('Ctrl Pts',(-0.282842712474619,1.6,4.28284271247462));
#9404=CARTESIAN_POINT('Ctrl Pts',(-0.278258894172667,1.58703500397985,4.28742653077657));
#9405=CARTESIAN_POINT('Ctrl Pts',(-0.274318439164033,1.57366719225041,4.29114637326852));
#9406=CARTESIAN_POINT('Ctrl Pts',(-0.266946656583193,1.5403635841556,4.2979507721165));
#9407=CARTESIAN_POINT('Ctrl Pts',(-0.264575131106459,1.52014467721507,4.3));
#9408=CARTESIAN_POINT('Ctrl Pts',(-0.264575131106459,1.5,4.3));
#9409=CARTESIAN_POINT('',(0.264575131106459,1.5,4.3));
#9410=CARTESIAN_POINT('Ctrl Pts',(0.264575131106459,1.5,4.3));
#9411=CARTESIAN_POINT('Ctrl Pts',(0.264575131106459,1.52014467721507,4.3));
#9412=CARTESIAN_POINT('Ctrl Pts',(0.266946656583193,1.5403635841556,4.2979507721165));
#9413=CARTESIAN_POINT('Ctrl Pts',(0.27431843921387,1.57366719247556,4.29114637322252));
#9414=CARTESIAN_POINT('Ctrl Pts',(0.278258894077422,1.58703500371046,4.28742653087182));
#9415=CARTESIAN_POINT('Ctrl Pts',(0.282842712474619,1.6,4.28284271247462));
#9416=CARTESIAN_POINT('',(0.282842712474619,1.6,3.71715728752538));
#9417=CARTESIAN_POINT('Ctrl Pts',(0.282842712474619,1.6,3.71715728752538));
#9418=CARTESIAN_POINT('Ctrl Pts',(0.278258894172666,1.58703500397985,3.71257346922343));
#9419=CARTESIAN_POINT('Ctrl Pts',(0.274318439164033,1.57366719225041,3.70885362673148));
#9420=CARTESIAN_POINT('Ctrl Pts',(0.266946656583194,1.5403635841556,3.7020492278835));
#9421=CARTESIAN_POINT('Ctrl Pts',(0.264575131106459,1.52014467721507,3.7));
#9422=CARTESIAN_POINT('Ctrl Pts',(0.264575131106459,1.5,3.7));
#9423=CARTESIAN_POINT('Ctrl Pts',(0.264575131106459,1.47985532278493,3.7));
#9424=CARTESIAN_POINT('Ctrl Pts',(0.266946656583194,1.4596364158444,3.7020492278835));
#9425=CARTESIAN_POINT('Ctrl Pts',(0.275663470560297,1.42025634008317,3.71009513514317));
#9426=CARTESIAN_POINT('Ctrl Pts',(0.281970270384708,1.40108570205275,3.71608711674642));
#9427=CARTESIAN_POINT('Ctrl Pts',(0.304063569802551,1.34650091982942,3.7392312552828));
#9428=CARTESIAN_POINT('Ctrl Pts',(0.322818652826944,1.31392187404012,3.76181405724795));
#9429=CARTESIAN_POINT('Ctrl Pts',(0.355071552231379,1.26236205014611,3.81337388114196));
#9430=CARTESIAN_POINT('Ctrl Pts',(0.371172434841458,1.23945139911714,3.84601764444721));
#9431=CARTESIAN_POINT('Ctrl Pts',(0.393713960479867,1.20823419970573,3.91957074694018));
#9432=CARTESIAN_POINT('Ctrl Pts',(0.4,1.2,3.96055805317426));
#9433=CARTESIAN_POINT('Ctrl Pts',(0.4,1.2,4.03944194682574));
#9434=CARTESIAN_POINT('Ctrl Pts',(0.393713960479867,1.20823419970573,4.08042925305982));
#9435=CARTESIAN_POINT('Ctrl Pts',(0.371172434841458,1.23945139911714,4.15398235555279));
#9436=CARTESIAN_POINT('Ctrl Pts',(0.35507155223138,1.26236205014611,4.18662611885804));
#9437=CARTESIAN_POINT('Ctrl Pts',(0.322818652826944,1.31392187404012,4.23818594275205));
#9438=CARTESIAN_POINT('Ctrl Pts',(0.304063569802551,1.34650091982942,4.2607687447172));
#9439=CARTESIAN_POINT('Ctrl Pts',(0.281970270384709,1.40108570205275,4.28391288325358));
#9440=CARTESIAN_POINT('Ctrl Pts',(0.275663470560297,1.42025634008317,4.28990486485683));
#9441=CARTESIAN_POINT('Ctrl Pts',(0.266946656583193,1.4596364158444,4.2979507721165));
#9442=CARTESIAN_POINT('Ctrl Pts',(0.264575131106459,1.47985532278493,4.3));
#9443=CARTESIAN_POINT('Ctrl Pts',(0.264575131106459,1.5,4.3));
#9444=CARTESIAN_POINT('',(-0.282842712474619,1.6,3.71715728752538));
#9445=CARTESIAN_POINT('Origin',(0.,1.6,4.));
#9446=CARTESIAN_POINT('Ctrl Pts',(-0.4,1.2,4.));
#9447=CARTESIAN_POINT('Ctrl Pts',(-0.4,1.2,3.96055805317426));
#9448=CARTESIAN_POINT('Ctrl Pts',(-0.393713960479867,1.20823419970573,3.91957074694018));
#9449=CARTESIAN_POINT('Ctrl Pts',(-0.371172434841458,1.23945139911714,3.84601764444721));
#9450=CARTESIAN_POINT('Ctrl Pts',(-0.355071552231379,1.26236205014611,3.81337388114196));
#9451=CARTESIAN_POINT('Ctrl Pts',(-0.322818652826944,1.31392187404012,3.76181405724795));
#9452=CARTESIAN_POINT('Ctrl Pts',(-0.30406356980255,1.34650091982942,3.7392312552828));
#9453=CARTESIAN_POINT('Ctrl Pts',(-0.281970270384708,1.40108570205275,3.71608711674642));
#9454=CARTESIAN_POINT('Ctrl Pts',(-0.275663470560297,1.42025634008317,3.71009513514317));
#9455=CARTESIAN_POINT('Ctrl Pts',(-0.266946656583194,1.4596364158444,3.7020492278835));
#9456=CARTESIAN_POINT('Ctrl Pts',(-0.264575131106459,1.47985532278493,3.7));
#9457=CARTESIAN_POINT('Ctrl Pts',(-0.264575131106459,1.5,3.7));
#9458=CARTESIAN_POINT('Ctrl Pts',(-0.264575131106459,1.52014467721507,3.7));
#9459=CARTESIAN_POINT('Ctrl Pts',(-0.266946656583194,1.5403635841556,3.7020492278835));
#9460=CARTESIAN_POINT('Ctrl Pts',(-0.27431843921387,1.57366719247556,3.70885362677748));
#9461=CARTESIAN_POINT('Ctrl Pts',(-0.278258894077422,1.58703500371046,3.71257346912818));
#9462=CARTESIAN_POINT('Ctrl Pts',(-0.282842712474619,1.6,3.71715728752538));
#9463=CARTESIAN_POINT('Origin',(0.,0.,4.));
#9464=CARTESIAN_POINT('Origin',(0.,-0.1,4.));
#9465=CARTESIAN_POINT('Origin',(0.,0.,4.));
#9466=CARTESIAN_POINT('Origin',(0.,0.,4.));
#9467=CARTESIAN_POINT('Origin',(0.,-0.1,4.));
#9468=CARTESIAN_POINT('',(-0.387298334620742,-0.1,4.1));
#9469=CARTESIAN_POINT('Origin',(0.,0.,4.));
#9470=CARTESIAN_POINT('Origin',(0.,-0.1,4.));
#9471=CARTESIAN_POINT('Origin',(0.,0.,4.));
#9472=CARTESIAN_POINT('Origin',(0.,1.6,4.));
#9473=CARTESIAN_POINT('',(-5.6,1.6,3.71715728752538));
#9474=CARTESIAN_POINT('Origin',(0.,-0.1,4.));
#9475=CARTESIAN_POINT('',(-0.387298334620742,-0.1,3.9));
#9476=CARTESIAN_POINT('Origin',(0.,0.,3.9));
#9477=CARTESIAN_POINT('Origin',(0.,0.,3.9));
#9478=CARTESIAN_POINT('Origin',(0.,0.,3.9));
#9479=CARTESIAN_POINT('Origin',(0.,0.,3.9));
#9480=CARTESIAN_POINT('Origin',(0.,0.,3.9));
#9481=CARTESIAN_POINT('Origin',(0.,0.,3.9));
#9482=CARTESIAN_POINT('',(-0.4,4.89858719658941E-17,4.6));
#9483=CARTESIAN_POINT('',(-0.4,-4.89858719658941E-17,3.9));
#9484=CARTESIAN_POINT('Origin',(0.,0.,4.6));
#9485=CARTESIAN_POINT('Origin',(0.,0.,3.9));
#9486=CARTESIAN_POINT('Origin',(0.,0.,3.9));
#9487=CARTESIAN_POINT('Origin',(0.,0.,3.9));
#9488=CARTESIAN_POINT('Origin',(0.,0.,4.6));
#9489=CARTESIAN_POINT('',(-0.685,-8.38883057415937E-17,4.6));
#9490=CARTESIAN_POINT('Origin',(0.,0.,4.6));
#9491=CARTESIAN_POINT('',(-0.685,8.38883057415937E-17,6.));
#9492=CARTESIAN_POINT('',(-0.685,-8.38883057415937E-17,4.6));
#9493=CARTESIAN_POINT('Origin',(0.,0.,6.));
#9494=CARTESIAN_POINT('Origin',(0.,0.,4.6));
#9495=CARTESIAN_POINT('Origin',(3.75,1.5,3.9));
#9496=CARTESIAN_POINT('',(3.75,1.35,4.25980762113533));
#9497=CARTESIAN_POINT('',(3.9,1.5,4.3));
#9498=CARTESIAN_POINT('Ctrl Pts',(3.75,1.35,4.25980762113533));
#9499=CARTESIAN_POINT('Ctrl Pts',(3.76924576004407,1.35,4.25980762113533));
#9500=CARTESIAN_POINT('Ctrl Pts',(3.78947079018949,1.35391716232849,4.26217381539294));
#9501=CARTESIAN_POINT('Ctrl Pts',(3.82628735392617,1.36931569353957,4.2701794018691));
#9502=CARTESIAN_POINT('Ctrl Pts',(3.84291866013631,1.38078662578034,4.27565507013233));
#9503=CARTESIAN_POINT('Ctrl Pts',(3.86917753388502,1.40704549952906,4.28557999151058));
#9504=CARTESIAN_POINT('Ctrl Pts',(3.88067476198869,1.42368888628284,4.29073972615592));
#9505=CARTESIAN_POINT('Ctrl Pts',(3.89609458588037,1.46055823867667,4.2979887952526));
#9506=CARTESIAN_POINT('Ctrl Pts',(3.9,1.4808067048337,4.3));
#9507=CARTESIAN_POINT('Ctrl Pts',(3.9,1.5,4.3));
#9508=CARTESIAN_POINT('',(3.6,1.5,4.3));
#9509=CARTESIAN_POINT('Ctrl Pts',(3.6,1.5,4.3));
#9510=CARTESIAN_POINT('Ctrl Pts',(3.6,1.4808067048337,4.3));
#9511=CARTESIAN_POINT('Ctrl Pts',(3.60390541411963,1.46055823867667,4.2979887952526));
#9512=CARTESIAN_POINT('Ctrl Pts',(3.61932523801131,1.42368888628284,4.29073972615592));
#9513=CARTESIAN_POINT('Ctrl Pts',(3.63082246611498,1.40704549952906,4.28557999151058));
#9514=CARTESIAN_POINT('Ctrl Pts',(3.65708133986369,1.38078662578034,4.27565507013233));
#9515=CARTESIAN_POINT('Ctrl Pts',(3.67371264607383,1.36931569353957,4.2701794018691));
#9516=CARTESIAN_POINT('Ctrl Pts',(3.71052920981051,1.35391716232849,4.26217381539294));
#9517=CARTESIAN_POINT('Ctrl Pts',(3.73075423995593,1.35,4.25980762113533));
#9518=CARTESIAN_POINT('Ctrl Pts',(3.75,1.35,4.25980762113533));
#9519=CARTESIAN_POINT('',(3.6,1.5,4.6));
#9520=CARTESIAN_POINT('',(3.6,1.5,3.9));
#9521=CARTESIAN_POINT('Origin',(3.75,1.5,4.6));
#9522=CARTESIAN_POINT('Ctrl Pts',(3.9,1.5,4.3));
#9523=CARTESIAN_POINT('Ctrl Pts',(3.9,1.5191932951663,4.3));
#9524=CARTESIAN_POINT('Ctrl Pts',(3.89609458588037,1.53944176132333,4.2979887952526));
#9525=CARTESIAN_POINT('Ctrl Pts',(3.88067476198869,1.57631111371716,4.29073972615592));
#9526=CARTESIAN_POINT('Ctrl Pts',(3.86917753388502,1.59295450047094,4.28557999151058));
#9527=CARTESIAN_POINT('Ctrl Pts',(3.84291866013631,1.61921337421966,4.27565507013233));
#9528=CARTESIAN_POINT('Ctrl Pts',(3.82628735392617,1.63068430646043,4.2701794018691));
#9529=CARTESIAN_POINT('Ctrl Pts',(3.78947079018949,1.64608283767151,4.26217381539294));
#9530=CARTESIAN_POINT('Ctrl Pts',(3.76924576004407,1.65,4.25980762113533));
#9531=CARTESIAN_POINT('Ctrl Pts',(3.73075423995593,1.65,4.25980762113533));
#9532=CARTESIAN_POINT('Ctrl Pts',(3.71052920981051,1.64608283767151,4.26217381539294));
#9533=CARTESIAN_POINT('Ctrl Pts',(3.67371264607383,1.63068430646043,4.2701794018691));
#9534=CARTESIAN_POINT('Ctrl Pts',(3.65708133986369,1.61921337421966,4.27565507013233));
#9535=CARTESIAN_POINT('Ctrl Pts',(3.63082246611498,1.59295450047094,4.28557999151058));
#9536=CARTESIAN_POINT('Ctrl Pts',(3.61932523801131,1.57631111371716,4.29073972615592));
#9537=CARTESIAN_POINT('Ctrl Pts',(3.60390541411963,1.53944176132333,4.2979887952526));
#9538=CARTESIAN_POINT('Ctrl Pts',(3.6,1.5191932951663,4.3));
#9539=CARTESIAN_POINT('Ctrl Pts',(3.6,1.5,4.3));
#9540=CARTESIAN_POINT('Origin',(3.75,1.5,4.6));
#9541=CARTESIAN_POINT('',(3.5,1.5,4.6));
#9542=CARTESIAN_POINT('Origin',(3.75,1.5,4.6));
#9543=CARTESIAN_POINT('',(3.5,1.5,6.));
#9544=CARTESIAN_POINT('',(3.5,1.5,4.6));
#9545=CARTESIAN_POINT('Origin',(3.75,1.5,6.));
#9546=CARTESIAN_POINT('Origin',(3.75,1.5,4.6));
#9547=CARTESIAN_POINT('Origin',(3.75,-1.9,4.));
#9548=CARTESIAN_POINT('',(3.55,-1.85,4.));
#9549=CARTESIAN_POINT('Origin',(3.75,-1.85,4.));
#9550=CARTESIAN_POINT('',(3.55,1.2,4.));
#9551=CARTESIAN_POINT('',(3.55,-1.9,4.));
#9552=CARTESIAN_POINT('',(3.75,1.27639320225002,4.2));
#9553=CARTESIAN_POINT('Ctrl Pts',(3.75,1.27639320225002,4.2));
#9554=CARTESIAN_POINT('Ctrl Pts',(3.72369817653558,1.27639320225002,4.2));
#9555=CARTESIAN_POINT('Ctrl Pts',(3.69666820397931,1.27127943107918,4.19456887761608));
#9556=CARTESIAN_POINT('Ctrl Pts',(3.64786664910034,1.25525524610686,4.17398313783528));
#9557=CARTESIAN_POINT('Ctrl Pts',(3.62597566474128,1.24472396775817,4.1588183772159));
#9558=CARTESIAN_POINT('Ctrl Pts',(3.59137301409757,1.22622807298917,4.12421572657219));
#9559=CARTESIAN_POINT('Ctrl Pts',(3.57608176712229,1.21683270447635,4.1022830144367));
#9560=CARTESIAN_POINT('Ctrl Pts',(3.55537554685969,1.20366430897624,4.05320424736513));
#9561=CARTESIAN_POINT('Ctrl Pts',(3.55,1.2,4.02601246699667));
#9562=CARTESIAN_POINT('Ctrl Pts',(3.55,1.2,4.));
#9563=CARTESIAN_POINT('Ctrl Pts',(3.55,1.2,4.));
#9564=CARTESIAN_POINT('Ctrl Pts',(3.55,1.2,3.97398753300333));
#9565=CARTESIAN_POINT('Ctrl Pts',(3.55537554685969,1.20366430897624,3.94679575263487));
#9566=CARTESIAN_POINT('Ctrl Pts',(3.57608176712229,1.21683270447635,3.8977169855633));
#9567=CARTESIAN_POINT('Ctrl Pts',(3.59137301409757,1.22622807298917,3.87578427342781));
#9568=CARTESIAN_POINT('Ctrl Pts',(3.62597566474128,1.24472396775817,3.8411816227841));
#9569=CARTESIAN_POINT('Ctrl Pts',(3.64786664910034,1.25525524610686,3.82601686216472));
#9570=CARTESIAN_POINT('Ctrl Pts',(3.69666820397931,1.27127943107918,3.80543112238393));
#9571=CARTESIAN_POINT('Ctrl Pts',(3.72369817653558,1.27639320225002,3.8));
#9572=CARTESIAN_POINT('Ctrl Pts',(3.77630182346442,1.27639320225002,3.8));
#9573=CARTESIAN_POINT('Ctrl Pts',(3.80333179602069,1.27127943107918,3.80543112238393));
#9574=CARTESIAN_POINT('Ctrl Pts',(3.85213335089966,1.25525524610686,3.82601686216472));
#9575=CARTESIAN_POINT('Ctrl Pts',(3.87402433525872,1.24472396775817,3.8411816227841));
#9576=CARTESIAN_POINT('Ctrl Pts',(3.90862698590243,1.22622807298917,3.87578427342781));
#9577=CARTESIAN_POINT('Ctrl Pts',(3.92391823287771,1.21683270447635,3.8977169855633));
#9578=CARTESIAN_POINT('Ctrl Pts',(3.94462445314031,1.20366430897624,3.94679575263487));
#9579=CARTESIAN_POINT('Ctrl Pts',(3.95,1.2,3.97398753300333));
#9580=CARTESIAN_POINT('Ctrl Pts',(3.95,1.2,4.02601246699667));
#9581=CARTESIAN_POINT('Ctrl Pts',(3.94462445314031,1.20366430897624,4.05320424736513));
#9582=CARTESIAN_POINT('Ctrl Pts',(3.92391823287771,1.21683270447635,4.1022830144367));
#9583=CARTESIAN_POINT('Ctrl Pts',(3.90862698590243,1.22622807298917,4.12421572657219));
#9584=CARTESIAN_POINT('Ctrl Pts',(3.87402433525872,1.24472396775817,4.1588183772159));
#9585=CARTESIAN_POINT('Ctrl Pts',(3.85213335089966,1.25525524610686,4.17398313783528));
#9586=CARTESIAN_POINT('Ctrl Pts',(3.80333179602069,1.27127943107918,4.19456887761608));
#9587=CARTESIAN_POINT('Ctrl Pts',(3.77630182346442,1.27639320225002,4.2));
#9588=CARTESIAN_POINT('Ctrl Pts',(3.75,1.27639320225002,4.2));
#9589=CARTESIAN_POINT('Origin',(3.75,-2.6,4.));
#9590=CARTESIAN_POINT('',(3.235,-2.5,4.));
#9591=CARTESIAN_POINT('Origin',(3.75,-2.5,4.));
#9592=CARTESIAN_POINT('',(3.235,-1.85,4.));
#9593=CARTESIAN_POINT('',(3.235,-2.6,4.));
#9594=CARTESIAN_POINT('Origin',(3.75,-1.85,4.));
#9595=CARTESIAN_POINT('Origin',(3.75,-1.85,4.));
#9596=CARTESIAN_POINT('Origin',(1.25,1.5,3.9));
#9597=CARTESIAN_POINT('',(1.25,1.35,4.25980762113533));
#9598=CARTESIAN_POINT('',(1.4,1.5,4.3));
#9599=CARTESIAN_POINT('Ctrl Pts',(1.25,1.35,4.25980762113533));
#9600=CARTESIAN_POINT('Ctrl Pts',(1.26924576004407,1.35,4.25980762113533));
#9601=CARTESIAN_POINT('Ctrl Pts',(1.28947079018949,1.35391716232849,4.26217381539294));
#9602=CARTESIAN_POINT('Ctrl Pts',(1.32628735392617,1.36931569353957,4.2701794018691));
#9603=CARTESIAN_POINT('Ctrl Pts',(1.34291866013631,1.38078662578034,4.27565507013233));
#9604=CARTESIAN_POINT('Ctrl Pts',(1.36917753388502,1.40704549952906,4.28557999151058));
#9605=CARTESIAN_POINT('Ctrl Pts',(1.38067476198869,1.42368888628284,4.29073972615592));
#9606=CARTESIAN_POINT('Ctrl Pts',(1.39609458588037,1.46055823867667,4.2979887952526));
#9607=CARTESIAN_POINT('Ctrl Pts',(1.4,1.4808067048337,4.3));
#9608=CARTESIAN_POINT('Ctrl Pts',(1.4,1.5,4.3));
#9609=CARTESIAN_POINT('',(1.1,1.5,4.3));
#9610=CARTESIAN_POINT('Ctrl Pts',(1.1,1.5,4.3));
#9611=CARTESIAN_POINT('Ctrl Pts',(1.1,1.4808067048337,4.3));
#9612=CARTESIAN_POINT('Ctrl Pts',(1.10390541411963,1.46055823867667,4.2979887952526));
#9613=CARTESIAN_POINT('Ctrl Pts',(1.11932523801131,1.42368888628284,4.29073972615592));
#9614=CARTESIAN_POINT('Ctrl Pts',(1.13082246611498,1.40704549952906,4.28557999151057));
#9615=CARTESIAN_POINT('Ctrl Pts',(1.15708133986369,1.38078662578034,4.27565507013233));
#9616=CARTESIAN_POINT('Ctrl Pts',(1.17371264607383,1.36931569353957,4.2701794018691));
#9617=CARTESIAN_POINT('Ctrl Pts',(1.21052920981051,1.35391716232849,4.26217381539294));
#9618=CARTESIAN_POINT('Ctrl Pts',(1.23075423995593,1.35,4.25980762113533));
#9619=CARTESIAN_POINT('Ctrl Pts',(1.25,1.35,4.25980762113533));
#9620=CARTESIAN_POINT('',(1.1,1.5,4.6));
#9621=CARTESIAN_POINT('',(1.1,1.5,3.9));
#9622=CARTESIAN_POINT('Origin',(1.25,1.5,4.6));
#9623=CARTESIAN_POINT('Ctrl Pts',(1.4,1.5,4.3));
#9624=CARTESIAN_POINT('Ctrl Pts',(1.4,1.5191932951663,4.3));
#9625=CARTESIAN_POINT('Ctrl Pts',(1.39609458588037,1.53944176132333,4.2979887952526));
#9626=CARTESIAN_POINT('Ctrl Pts',(1.38067476198869,1.57631111371716,4.29073972615592));
#9627=CARTESIAN_POINT('Ctrl Pts',(1.36917753388502,1.59295450047094,4.28557999151058));
#9628=CARTESIAN_POINT('Ctrl Pts',(1.34291866013631,1.61921337421966,4.27565507013233));
#9629=CARTESIAN_POINT('Ctrl Pts',(1.32628735392617,1.63068430646043,4.2701794018691));
#9630=CARTESIAN_POINT('Ctrl Pts',(1.28947079018949,1.64608283767151,4.26217381539294));
#9631=CARTESIAN_POINT('Ctrl Pts',(1.26924576004407,1.65,4.25980762113533));
#9632=CARTESIAN_POINT('Ctrl Pts',(1.23075423995593,1.65,4.25980762113533));
#9633=CARTESIAN_POINT('Ctrl Pts',(1.21052920981051,1.64608283767151,4.26217381539294));
#9634=CARTESIAN_POINT('Ctrl Pts',(1.17371264607383,1.63068430646043,4.2701794018691));
#9635=CARTESIAN_POINT('Ctrl Pts',(1.15708133986369,1.61921337421966,4.27565507013233));
#9636=CARTESIAN_POINT('Ctrl Pts',(1.13082246611498,1.59295450047094,4.28557999151058));
#9637=CARTESIAN_POINT('Ctrl Pts',(1.11932523801131,1.57631111371716,4.29073972615592));
#9638=CARTESIAN_POINT('Ctrl Pts',(1.10390541411963,1.53944176132333,4.2979887952526));
#9639=CARTESIAN_POINT('Ctrl Pts',(1.1,1.5191932951663,4.3));
#9640=CARTESIAN_POINT('Ctrl Pts',(1.1,1.5,4.3));
#9641=CARTESIAN_POINT('Origin',(1.25,1.5,4.6));
#9642=CARTESIAN_POINT('',(1.,1.5,4.6));
#9643=CARTESIAN_POINT('Origin',(1.25,1.5,4.6));
#9644=CARTESIAN_POINT('',(1.,1.5,6.));
#9645=CARTESIAN_POINT('',(1.,1.5,4.6));
#9646=CARTESIAN_POINT('Origin',(1.25,1.5,6.));
#9647=CARTESIAN_POINT('Origin',(1.25,1.5,4.6));
#9648=CARTESIAN_POINT('Origin',(1.25,-1.9,4.));
#9649=CARTESIAN_POINT('',(1.05,-1.85,4.));
#9650=CARTESIAN_POINT('Origin',(1.25,-1.85,4.));
#9651=CARTESIAN_POINT('',(1.05,1.2,4.));
#9652=CARTESIAN_POINT('',(1.05,-1.9,4.));
#9653=CARTESIAN_POINT('',(1.25,1.27639320225002,4.2));
#9654=CARTESIAN_POINT('Ctrl Pts',(1.25,1.27639320225002,4.2));
#9655=CARTESIAN_POINT('Ctrl Pts',(1.22369817653558,1.27639320225002,4.2));
#9656=CARTESIAN_POINT('Ctrl Pts',(1.19666820397931,1.27127943107918,4.19456887761608));
#9657=CARTESIAN_POINT('Ctrl Pts',(1.14786664910035,1.25525524610686,4.17398313783528));
#9658=CARTESIAN_POINT('Ctrl Pts',(1.12597566474129,1.24472396775817,4.1588183772159));
#9659=CARTESIAN_POINT('Ctrl Pts',(1.09137301409758,1.22622807298917,4.12421572657219));
#9660=CARTESIAN_POINT('Ctrl Pts',(1.07608176712229,1.21683270447635,4.1022830144367));
#9661=CARTESIAN_POINT('Ctrl Pts',(1.05537554685969,1.20366430897624,4.05320424736513));
#9662=CARTESIAN_POINT('Ctrl Pts',(1.05,1.2,4.02601246699667));
#9663=CARTESIAN_POINT('Ctrl Pts',(1.05,1.2,4.));
#9664=CARTESIAN_POINT('Ctrl Pts',(1.05,1.2,4.));
#9665=CARTESIAN_POINT('Ctrl Pts',(1.05,1.2,3.97398753300333));
#9666=CARTESIAN_POINT('Ctrl Pts',(1.05537554685969,1.20366430897624,3.94679575263487));
#9667=CARTESIAN_POINT('Ctrl Pts',(1.07608176712229,1.21683270447635,3.8977169855633));
#9668=CARTESIAN_POINT('Ctrl Pts',(1.09137301409758,1.22622807298917,3.87578427342781));
#9669=CARTESIAN_POINT('Ctrl Pts',(1.12597566474129,1.24472396775817,3.8411816227841));
#9670=CARTESIAN_POINT('Ctrl Pts',(1.14786664910034,1.25525524610686,3.82601686216472));
#9671=CARTESIAN_POINT('Ctrl Pts',(1.19666820397931,1.27127943107918,3.80543112238393));
#9672=CARTESIAN_POINT('Ctrl Pts',(1.22369817653558,1.27639320225002,3.8));
#9673=CARTESIAN_POINT('Ctrl Pts',(1.27630182346442,1.27639320225002,3.8));
#9674=CARTESIAN_POINT('Ctrl Pts',(1.30333179602069,1.27127943107918,3.80543112238393));
#9675=CARTESIAN_POINT('Ctrl Pts',(1.35213335089966,1.25525524610686,3.82601686216472));
#9676=CARTESIAN_POINT('Ctrl Pts',(1.37402433525871,1.24472396775817,3.8411816227841));
#9677=CARTESIAN_POINT('Ctrl Pts',(1.40862698590242,1.22622807298917,3.87578427342781));
#9678=CARTESIAN_POINT('Ctrl Pts',(1.42391823287771,1.21683270447635,3.8977169855633));
#9679=CARTESIAN_POINT('Ctrl Pts',(1.44462445314031,1.20366430897624,3.94679575263487));
#9680=CARTESIAN_POINT('Ctrl Pts',(1.45,1.2,3.97398753300333));
#9681=CARTESIAN_POINT('Ctrl Pts',(1.45,1.2,4.02601246699667));
#9682=CARTESIAN_POINT('Ctrl Pts',(1.44462445314031,1.20366430897624,4.05320424736513));
#9683=CARTESIAN_POINT('Ctrl Pts',(1.42391823287771,1.21683270447635,4.1022830144367));
#9684=CARTESIAN_POINT('Ctrl Pts',(1.40862698590242,1.22622807298917,4.12421572657219));
#9685=CARTESIAN_POINT('Ctrl Pts',(1.37402433525871,1.24472396775817,4.1588183772159));
#9686=CARTESIAN_POINT('Ctrl Pts',(1.35213335089966,1.25525524610686,4.17398313783528));
#9687=CARTESIAN_POINT('Ctrl Pts',(1.30333179602069,1.27127943107918,4.19456887761608));
#9688=CARTESIAN_POINT('Ctrl Pts',(1.27630182346442,1.27639320225002,4.2));
#9689=CARTESIAN_POINT('Ctrl Pts',(1.25,1.27639320225002,4.2));
#9690=CARTESIAN_POINT('Origin',(1.25,-2.6,4.));
#9691=CARTESIAN_POINT('',(0.735,-2.5,4.));
#9692=CARTESIAN_POINT('Origin',(1.25,-2.5,4.));
#9693=CARTESIAN_POINT('',(0.735,-1.85,4.));
#9694=CARTESIAN_POINT('',(0.735,-2.6,4.));
#9695=CARTESIAN_POINT('Origin',(1.25,-1.85,4.));
#9696=CARTESIAN_POINT('Origin',(1.25,-1.85,4.));
#9697=CARTESIAN_POINT('Origin',(-1.25,1.5,3.9));
#9698=CARTESIAN_POINT('',(-1.25,1.35,4.25980762113533));
#9699=CARTESIAN_POINT('',(-1.1,1.5,4.3));
#9700=CARTESIAN_POINT('Ctrl Pts',(-1.25,1.35,4.25980762113533));
#9701=CARTESIAN_POINT('Ctrl Pts',(-1.23075423995593,1.35,4.25980762113533));
#9702=CARTESIAN_POINT('Ctrl Pts',(-1.21052920981051,1.35391716232849,4.26217381539294));
#9703=CARTESIAN_POINT('Ctrl Pts',(-1.17371264607383,1.36931569353957,4.2701794018691));
#9704=CARTESIAN_POINT('Ctrl Pts',(-1.15708133986369,1.38078662578034,4.27565507013233));
#9705=CARTESIAN_POINT('Ctrl Pts',(-1.13082246611498,1.40704549952906,4.28557999151058));
#9706=CARTESIAN_POINT('Ctrl Pts',(-1.11932523801131,1.42368888628284,4.29073972615592));
#9707=CARTESIAN_POINT('Ctrl Pts',(-1.10390541411963,1.46055823867667,4.2979887952526));
#9708=CARTESIAN_POINT('Ctrl Pts',(-1.1,1.4808067048337,4.3));
#9709=CARTESIAN_POINT('Ctrl Pts',(-1.1,1.5,4.3));
#9710=CARTESIAN_POINT('',(-1.4,1.5,4.3));
#9711=CARTESIAN_POINT('Ctrl Pts',(-1.4,1.5,4.3));
#9712=CARTESIAN_POINT('Ctrl Pts',(-1.4,1.4808067048337,4.3));
#9713=CARTESIAN_POINT('Ctrl Pts',(-1.39609458588037,1.46055823867667,4.2979887952526));
#9714=CARTESIAN_POINT('Ctrl Pts',(-1.38067476198869,1.42368888628284,4.29073972615592));
#9715=CARTESIAN_POINT('Ctrl Pts',(-1.36917753388502,1.40704549952906,4.28557999151058));
#9716=CARTESIAN_POINT('Ctrl Pts',(-1.34291866013631,1.38078662578034,4.27565507013233));
#9717=CARTESIAN_POINT('Ctrl Pts',(-1.32628735392617,1.36931569353957,4.2701794018691));
#9718=CARTESIAN_POINT('Ctrl Pts',(-1.28947079018949,1.35391716232849,4.26217381539294));
#9719=CARTESIAN_POINT('Ctrl Pts',(-1.26924576004407,1.35,4.25980762113533));
#9720=CARTESIAN_POINT('Ctrl Pts',(-1.25,1.35,4.25980762113533));
#9721=CARTESIAN_POINT('',(-1.4,1.5,4.6));
#9722=CARTESIAN_POINT('',(-1.4,1.5,3.9));
#9723=CARTESIAN_POINT('Origin',(-1.25,1.5,4.6));
#9724=CARTESIAN_POINT('Ctrl Pts',(-1.1,1.5,4.3));
#9725=CARTESIAN_POINT('Ctrl Pts',(-1.1,1.5191932951663,4.3));
#9726=CARTESIAN_POINT('Ctrl Pts',(-1.10390541411963,1.53944176132333,4.2979887952526));
#9727=CARTESIAN_POINT('Ctrl Pts',(-1.11932523801131,1.57631111371716,4.29073972615592));
#9728=CARTESIAN_POINT('Ctrl Pts',(-1.13082246611498,1.59295450047094,4.28557999151058));
#9729=CARTESIAN_POINT('Ctrl Pts',(-1.15708133986369,1.61921337421966,4.27565507013233));
#9730=CARTESIAN_POINT('Ctrl Pts',(-1.17371264607383,1.63068430646043,4.2701794018691));
#9731=CARTESIAN_POINT('Ctrl Pts',(-1.21052920981051,1.64608283767151,4.26217381539294));
#9732=CARTESIAN_POINT('Ctrl Pts',(-1.23075423995593,1.65,4.25980762113533));
#9733=CARTESIAN_POINT('Ctrl Pts',(-1.26924576004407,1.65,4.25980762113533));
#9734=CARTESIAN_POINT('Ctrl Pts',(-1.28947079018949,1.64608283767151,4.26217381539294));
#9735=CARTESIAN_POINT('Ctrl Pts',(-1.32628735392617,1.63068430646043,4.2701794018691));
#9736=CARTESIAN_POINT('Ctrl Pts',(-1.34291866013631,1.61921337421966,4.27565507013233));
#9737=CARTESIAN_POINT('Ctrl Pts',(-1.36917753388502,1.59295450047094,4.28557999151058));
#9738=CARTESIAN_POINT('Ctrl Pts',(-1.38067476198869,1.57631111371716,4.29073972615592));
#9739=CARTESIAN_POINT('Ctrl Pts',(-1.39609458588037,1.53944176132333,4.2979887952526));
#9740=CARTESIAN_POINT('Ctrl Pts',(-1.4,1.5191932951663,4.3));
#9741=CARTESIAN_POINT('Ctrl Pts',(-1.4,1.5,4.3));
#9742=CARTESIAN_POINT('Origin',(-1.25,1.5,4.6));
#9743=CARTESIAN_POINT('',(-1.5,1.5,4.6));
#9744=CARTESIAN_POINT('Origin',(-1.25,1.5,4.6));
#9745=CARTESIAN_POINT('',(-1.5,1.5,6.));
#9746=CARTESIAN_POINT('',(-1.5,1.5,4.6));
#9747=CARTESIAN_POINT('Origin',(-1.25,1.5,6.));
#9748=CARTESIAN_POINT('Origin',(-1.25,1.5,4.6));
#9749=CARTESIAN_POINT('Origin',(-1.25,-1.9,4.));
#9750=CARTESIAN_POINT('',(-1.45,-1.85,4.));
#9751=CARTESIAN_POINT('Origin',(-1.25,-1.85,4.));
#9752=CARTESIAN_POINT('',(-1.45,1.2,4.));
#9753=CARTESIAN_POINT('',(-1.45,-1.9,4.));
#9754=CARTESIAN_POINT('',(-1.25,1.27639320225002,4.2));
#9755=CARTESIAN_POINT('Ctrl Pts',(-1.25,1.27639320225002,4.2));
#9756=CARTESIAN_POINT('Ctrl Pts',(-1.27630182346442,1.27639320225002,4.2));
#9757=CARTESIAN_POINT('Ctrl Pts',(-1.30333179602069,1.27127943107918,4.19456887761608));
#9758=CARTESIAN_POINT('Ctrl Pts',(-1.35213335089965,1.25525524610686,4.17398313783528));
#9759=CARTESIAN_POINT('Ctrl Pts',(-1.37402433525871,1.24472396775817,4.1588183772159));
#9760=CARTESIAN_POINT('Ctrl Pts',(-1.40862698590242,1.22622807298917,4.12421572657219));
#9761=CARTESIAN_POINT('Ctrl Pts',(-1.42391823287771,1.21683270447635,4.1022830144367));
#9762=CARTESIAN_POINT('Ctrl Pts',(-1.44462445314031,1.20366430897624,4.05320424736513));
#9763=CARTESIAN_POINT('Ctrl Pts',(-1.45,1.2,4.02601246699667));
#9764=CARTESIAN_POINT('Ctrl Pts',(-1.45,1.2,4.));
#9765=CARTESIAN_POINT('Ctrl Pts',(-1.45,1.2,4.));
#9766=CARTESIAN_POINT('Ctrl Pts',(-1.45,1.2,3.97398753300333));
#9767=CARTESIAN_POINT('Ctrl Pts',(-1.44462445314031,1.20366430897624,3.94679575263487));
#9768=CARTESIAN_POINT('Ctrl Pts',(-1.42391823287771,1.21683270447635,3.8977169855633));
#9769=CARTESIAN_POINT('Ctrl Pts',(-1.40862698590242,1.22622807298917,3.87578427342781));
#9770=CARTESIAN_POINT('Ctrl Pts',(-1.37402433525871,1.24472396775817,3.8411816227841));
#9771=CARTESIAN_POINT('Ctrl Pts',(-1.35213335089966,1.25525524610686,3.82601686216472));
#9772=CARTESIAN_POINT('Ctrl Pts',(-1.30333179602069,1.27127943107918,3.80543112238392));
#9773=CARTESIAN_POINT('Ctrl Pts',(-1.27630182346442,1.27639320225002,3.8));
#9774=CARTESIAN_POINT('Ctrl Pts',(-1.22369817653558,1.27639320225002,3.8));
#9775=CARTESIAN_POINT('Ctrl Pts',(-1.19666820397931,1.27127943107918,3.80543112238393));
#9776=CARTESIAN_POINT('Ctrl Pts',(-1.14786664910034,1.25525524610686,3.82601686216472));
#9777=CARTESIAN_POINT('Ctrl Pts',(-1.12597566474129,1.24472396775817,3.8411816227841));
#9778=CARTESIAN_POINT('Ctrl Pts',(-1.09137301409758,1.22622807298917,3.87578427342781));
#9779=CARTESIAN_POINT('Ctrl Pts',(-1.07608176712229,1.21683270447635,3.8977169855633));
#9780=CARTESIAN_POINT('Ctrl Pts',(-1.05537554685969,1.20366430897624,3.94679575263487));
#9781=CARTESIAN_POINT('Ctrl Pts',(-1.05,1.2,3.97398753300333));
#9782=CARTESIAN_POINT('Ctrl Pts',(-1.05,1.2,4.02601246699667));
#9783=CARTESIAN_POINT('Ctrl Pts',(-1.05537554685969,1.20366430897624,4.05320424736513));
#9784=CARTESIAN_POINT('Ctrl Pts',(-1.07608176712229,1.21683270447635,4.10228301443669));
#9785=CARTESIAN_POINT('Ctrl Pts',(-1.09137301409758,1.22622807298917,4.12421572657219));
#9786=CARTESIAN_POINT('Ctrl Pts',(-1.12597566474129,1.24472396775817,4.1588183772159));
#9787=CARTESIAN_POINT('Ctrl Pts',(-1.14786664910034,1.25525524610686,4.17398313783528));
#9788=CARTESIAN_POINT('Ctrl Pts',(-1.19666820397931,1.27127943107918,4.19456887761607));
#9789=CARTESIAN_POINT('Ctrl Pts',(-1.22369817653558,1.27639320225002,4.2));
#9790=CARTESIAN_POINT('Ctrl Pts',(-1.25,1.27639320225002,4.2));
#9791=CARTESIAN_POINT('Origin',(-1.25,-2.6,4.));
#9792=CARTESIAN_POINT('',(-1.765,-2.5,4.));
#9793=CARTESIAN_POINT('Origin',(-1.25,-2.5,4.));
#9794=CARTESIAN_POINT('',(-1.765,-1.85,4.));
#9795=CARTESIAN_POINT('',(-1.765,-2.6,4.));
#9796=CARTESIAN_POINT('Origin',(-1.25,-1.85,4.));
#9797=CARTESIAN_POINT('Origin',(-1.25,-1.85,4.));
#9798=CARTESIAN_POINT('Origin',(-3.75,1.5,3.9));
#9799=CARTESIAN_POINT('',(-3.75,1.35,4.25980762113533));
#9800=CARTESIAN_POINT('',(-3.6,1.5,4.3));
#9801=CARTESIAN_POINT('Ctrl Pts',(-3.75,1.35,4.25980762113533));
#9802=CARTESIAN_POINT('Ctrl Pts',(-3.73075423995593,1.35,4.25980762113533));
#9803=CARTESIAN_POINT('Ctrl Pts',(-3.71052920981051,1.35391716232849,4.26217381539294));
#9804=CARTESIAN_POINT('Ctrl Pts',(-3.67371264607383,1.36931569353957,4.2701794018691));
#9805=CARTESIAN_POINT('Ctrl Pts',(-3.65708133986369,1.38078662578034,4.27565507013233));
#9806=CARTESIAN_POINT('Ctrl Pts',(-3.63082246611498,1.40704549952906,4.28557999151058));
#9807=CARTESIAN_POINT('Ctrl Pts',(-3.61932523801131,1.42368888628284,4.29073972615592));
#9808=CARTESIAN_POINT('Ctrl Pts',(-3.60390541411963,1.46055823867667,4.2979887952526));
#9809=CARTESIAN_POINT('Ctrl Pts',(-3.6,1.4808067048337,4.3));
#9810=CARTESIAN_POINT('Ctrl Pts',(-3.6,1.5,4.3));
#9811=CARTESIAN_POINT('',(-3.9,1.5,4.3));
#9812=CARTESIAN_POINT('Ctrl Pts',(-3.9,1.5,4.3));
#9813=CARTESIAN_POINT('Ctrl Pts',(-3.9,1.4808067048337,4.3));
#9814=CARTESIAN_POINT('Ctrl Pts',(-3.89609458588037,1.46055823867667,4.2979887952526));
#9815=CARTESIAN_POINT('Ctrl Pts',(-3.88067476198869,1.42368888628284,4.29073972615592));
#9816=CARTESIAN_POINT('Ctrl Pts',(-3.86917753388502,1.40704549952906,4.28557999151058));
#9817=CARTESIAN_POINT('Ctrl Pts',(-3.84291866013631,1.38078662578034,4.27565507013233));
#9818=CARTESIAN_POINT('Ctrl Pts',(-3.82628735392617,1.36931569353957,4.2701794018691));
#9819=CARTESIAN_POINT('Ctrl Pts',(-3.78947079018949,1.35391716232849,4.26217381539294));
#9820=CARTESIAN_POINT('Ctrl Pts',(-3.76924576004407,1.35,4.25980762113533));
#9821=CARTESIAN_POINT('Ctrl Pts',(-3.75,1.35,4.25980762113533));
#9822=CARTESIAN_POINT('',(-3.9,1.5,4.6));
#9823=CARTESIAN_POINT('',(-3.9,1.5,3.9));
#9824=CARTESIAN_POINT('Origin',(-3.75,1.5,4.6));
#9825=CARTESIAN_POINT('Ctrl Pts',(-3.6,1.5,4.3));
#9826=CARTESIAN_POINT('Ctrl Pts',(-3.6,1.5191932951663,4.3));
#9827=CARTESIAN_POINT('Ctrl Pts',(-3.60390541411963,1.53944176132333,4.2979887952526));
#9828=CARTESIAN_POINT('Ctrl Pts',(-3.61932523801131,1.57631111371716,4.29073972615592));
#9829=CARTESIAN_POINT('Ctrl Pts',(-3.63082246611498,1.59295450047094,4.28557999151058));
#9830=CARTESIAN_POINT('Ctrl Pts',(-3.65708133986369,1.61921337421966,4.27565507013233));
#9831=CARTESIAN_POINT('Ctrl Pts',(-3.67371264607383,1.63068430646043,4.2701794018691));
#9832=CARTESIAN_POINT('Ctrl Pts',(-3.71052920981051,1.64608283767151,4.26217381539294));
#9833=CARTESIAN_POINT('Ctrl Pts',(-3.73075423995593,1.65,4.25980762113533));
#9834=CARTESIAN_POINT('Ctrl Pts',(-3.76924576004407,1.65,4.25980762113533));
#9835=CARTESIAN_POINT('Ctrl Pts',(-3.78947079018949,1.64608283767151,4.26217381539294));
#9836=CARTESIAN_POINT('Ctrl Pts',(-3.82628735392617,1.63068430646043,4.2701794018691));
#9837=CARTESIAN_POINT('Ctrl Pts',(-3.84291866013631,1.61921337421966,4.27565507013233));
#9838=CARTESIAN_POINT('Ctrl Pts',(-3.86917753388502,1.59295450047094,4.28557999151058));
#9839=CARTESIAN_POINT('Ctrl Pts',(-3.88067476198869,1.57631111371716,4.29073972615592));
#9840=CARTESIAN_POINT('Ctrl Pts',(-3.89609458588037,1.53944176132333,4.2979887952526));
#9841=CARTESIAN_POINT('Ctrl Pts',(-3.9,1.5191932951663,4.3));
#9842=CARTESIAN_POINT('Ctrl Pts',(-3.9,1.5,4.3));
#9843=CARTESIAN_POINT('Origin',(-3.75,1.5,4.6));
#9844=CARTESIAN_POINT('',(-4.,1.5,4.6));
#9845=CARTESIAN_POINT('Origin',(-3.75,1.5,4.6));
#9846=CARTESIAN_POINT('',(-4.,1.5,6.));
#9847=CARTESIAN_POINT('',(-4.,1.5,4.6));
#9848=CARTESIAN_POINT('Origin',(-3.75,1.5,6.));
#9849=CARTESIAN_POINT('Origin',(-3.75,1.5,4.6));
#9850=CARTESIAN_POINT('Origin',(-3.75,-1.9,4.));
#9851=CARTESIAN_POINT('',(-3.95,-1.85,4.));
#9852=CARTESIAN_POINT('Origin',(-3.75,-1.85,4.));
#9853=CARTESIAN_POINT('',(-3.95,1.2,4.));
#9854=CARTESIAN_POINT('',(-3.95,-1.9,4.));
#9855=CARTESIAN_POINT('',(-3.75,1.27639320225002,4.2));
#9856=CARTESIAN_POINT('Ctrl Pts',(-3.75,1.27639320225002,4.2));
#9857=CARTESIAN_POINT('Ctrl Pts',(-3.77630182346442,1.27639320225002,4.2));
#9858=CARTESIAN_POINT('Ctrl Pts',(-3.80333179602069,1.27127943107918,4.19456887761608));
#9859=CARTESIAN_POINT('Ctrl Pts',(-3.85213335089966,1.25525524610686,4.17398313783528));
#9860=CARTESIAN_POINT('Ctrl Pts',(-3.87402433525872,1.24472396775817,4.1588183772159));
#9861=CARTESIAN_POINT('Ctrl Pts',(-3.90862698590243,1.22622807298917,4.12421572657219));
#9862=CARTESIAN_POINT('Ctrl Pts',(-3.92391823287771,1.21683270447635,4.1022830144367));
#9863=CARTESIAN_POINT('Ctrl Pts',(-3.94462445314031,1.20366430897624,4.05320424736513));
#9864=CARTESIAN_POINT('Ctrl Pts',(-3.95,1.2,4.02601246699667));
#9865=CARTESIAN_POINT('Ctrl Pts',(-3.95,1.2,4.));
#9866=CARTESIAN_POINT('Ctrl Pts',(-3.95,1.2,4.));
#9867=CARTESIAN_POINT('Ctrl Pts',(-3.95,1.2,3.97398753300333));
#9868=CARTESIAN_POINT('Ctrl Pts',(-3.94462445314031,1.20366430897624,3.94679575263487));
#9869=CARTESIAN_POINT('Ctrl Pts',(-3.92391823287771,1.21683270447635,3.8977169855633));
#9870=CARTESIAN_POINT('Ctrl Pts',(-3.90862698590243,1.22622807298917,3.87578427342781));
#9871=CARTESIAN_POINT('Ctrl Pts',(-3.87402433525872,1.24472396775817,3.8411816227841));
#9872=CARTESIAN_POINT('Ctrl Pts',(-3.85213335089965,1.25525524610686,3.82601686216472));
#9873=CARTESIAN_POINT('Ctrl Pts',(-3.80333179602069,1.27127943107918,3.80543112238392));
#9874=CARTESIAN_POINT('Ctrl Pts',(-3.77630182346442,1.27639320225002,3.8));
#9875=CARTESIAN_POINT('Ctrl Pts',(-3.72369817653558,1.27639320225002,3.8));
#9876=CARTESIAN_POINT('Ctrl Pts',(-3.69666820397931,1.27127943107918,3.80543112238392));
#9877=CARTESIAN_POINT('Ctrl Pts',(-3.64786664910034,1.25525524610686,3.82601686216472));
#9878=CARTESIAN_POINT('Ctrl Pts',(-3.62597566474128,1.24472396775817,3.8411816227841));
#9879=CARTESIAN_POINT('Ctrl Pts',(-3.59137301409757,1.22622807298917,3.87578427342781));
#9880=CARTESIAN_POINT('Ctrl Pts',(-3.57608176712229,1.21683270447635,3.8977169855633));
#9881=CARTESIAN_POINT('Ctrl Pts',(-3.55537554685969,1.20366430897624,3.94679575263487));
#9882=CARTESIAN_POINT('Ctrl Pts',(-3.55,1.2,3.97398753300333));
#9883=CARTESIAN_POINT('Ctrl Pts',(-3.55,1.2,4.02601246699667));
#9884=CARTESIAN_POINT('Ctrl Pts',(-3.55537554685969,1.20366430897624,4.05320424736513));
#9885=CARTESIAN_POINT('Ctrl Pts',(-3.57608176712229,1.21683270447635,4.1022830144367));
#9886=CARTESIAN_POINT('Ctrl Pts',(-3.59137301409757,1.22622807298917,4.12421572657219));
#9887=CARTESIAN_POINT('Ctrl Pts',(-3.62597566474128,1.24472396775817,4.1588183772159));
#9888=CARTESIAN_POINT('Ctrl Pts',(-3.64786664910034,1.25525524610686,4.17398313783528));
#9889=CARTESIAN_POINT('Ctrl Pts',(-3.69666820397931,1.27127943107918,4.19456887761607));
#9890=CARTESIAN_POINT('Ctrl Pts',(-3.72369817653558,1.27639320225002,4.2));
#9891=CARTESIAN_POINT('Ctrl Pts',(-3.75,1.27639320225002,4.2));
#9892=CARTESIAN_POINT('Origin',(-3.75,-2.6,4.));
#9893=CARTESIAN_POINT('',(-4.265,-2.5,4.));
#9894=CARTESIAN_POINT('Origin',(-3.75,-2.5,4.));
#9895=CARTESIAN_POINT('',(-4.265,-1.85,4.));
#9896=CARTESIAN_POINT('',(-4.265,-2.6,4.));
#9897=CARTESIAN_POINT('Origin',(-3.75,-1.85,4.));
#9898=CARTESIAN_POINT('Origin',(-3.75,-1.85,4.));
#9899=CARTESIAN_POINT('Origin',(-5.6,1.5,4.));
#9900=CARTESIAN_POINT('',(-5.5,1.5,4.3));
#9901=CARTESIAN_POINT('Origin',(-5.5,1.5,4.));
#9902=CARTESIAN_POINT('',(-5.6,1.5,4.3));
#9903=CARTESIAN_POINT('',(-5.6,1.5,4.3));
#9904=CARTESIAN_POINT('',(-5.6,1.5,4.3));
#9905=CARTESIAN_POINT('',(-5.6,1.5,4.3));
#9906=CARTESIAN_POINT('',(-5.6,1.5,4.3));
#9907=CARTESIAN_POINT('',(5.5,1.5,4.3));
#9908=CARTESIAN_POINT('',(-5.6,1.5,4.3));
#9909=CARTESIAN_POINT('Origin',(5.5,1.5,4.));
#9910=CARTESIAN_POINT('Origin',(4.8,-1.8,3.8));
#9911=CARTESIAN_POINT('',(4.4,-1.8,3.8));
#9912=CARTESIAN_POINT('Origin',(4.8,-1.8,3.8));
#9913=CARTESIAN_POINT('',(4.4,-1.8,6.));
#9914=CARTESIAN_POINT('',(4.4,-1.8,3.8));
#9915=CARTESIAN_POINT('Origin',(4.8,-1.8,6.));
#9916=CARTESIAN_POINT('Origin',(4.8,-1.8,3.8));
#9917=CARTESIAN_POINT('',(4.575,-1.8,3.8));
#9918=CARTESIAN_POINT('Origin',(4.8,-1.8,3.8));
#9919=CARTESIAN_POINT('Origin',(-4.8,0.,3.8));
#9920=CARTESIAN_POINT('',(-5.2,-4.89858719658942E-17,3.8));
#9921=CARTESIAN_POINT('Origin',(-4.8,0.,3.8));
#9922=CARTESIAN_POINT('',(-5.2,4.89858719658942E-17,6.));
#9923=CARTESIAN_POINT('',(-5.2,-4.89858719658942E-17,3.8));
#9924=CARTESIAN_POINT('Origin',(-4.8,0.,6.));
#9925=CARTESIAN_POINT('Origin',(-4.8,0.,3.8));
#9926=CARTESIAN_POINT('',(-5.025,-2.75545529808154E-17,3.8));
#9927=CARTESIAN_POINT('Origin',(-4.8,0.,3.8));
#9928=CARTESIAN_POINT('Origin',(-4.8,-1.8,3.8));
#9929=CARTESIAN_POINT('',(-5.2,-1.8,3.8));
#9930=CARTESIAN_POINT('Origin',(-4.8,-1.8,3.8));
#9931=CARTESIAN_POINT('',(-5.2,-1.8,6.));
#9932=CARTESIAN_POINT('',(-5.2,-1.8,3.8));
#9933=CARTESIAN_POINT('Origin',(-4.8,-1.8,6.));
#9934=CARTESIAN_POINT('Origin',(-4.8,-1.8,3.8));
#9935=CARTESIAN_POINT('',(-5.025,-1.8,3.8));
#9936=CARTESIAN_POINT('Origin',(-4.8,-1.8,3.8));
#9937=CARTESIAN_POINT('Origin',(4.8,0.,3.8));
#9938=CARTESIAN_POINT('',(4.4,-4.89858719658942E-17,3.8));
#9939=CARTESIAN_POINT('Origin',(4.8,0.,3.8));
#9940=CARTESIAN_POINT('',(4.4,4.89858719658942E-17,6.));
#9941=CARTESIAN_POINT('',(4.4,-4.89858719658942E-17,3.8));
#9942=CARTESIAN_POINT('Origin',(4.8,0.,6.));
#9943=CARTESIAN_POINT('Origin',(4.8,0.,3.8));
#9944=CARTESIAN_POINT('',(4.575,-2.75545529808154E-17,3.8));
#9945=CARTESIAN_POINT('Origin',(4.8,0.,3.8));
#9946=CARTESIAN_POINT('Origin',(4.8,-1.8,2.9));
#9947=CARTESIAN_POINT('',(4.575,-1.8,3.));
#9948=CARTESIAN_POINT('Origin',(4.8,-1.8,3.));
#9949=CARTESIAN_POINT('',(4.575,-1.8,2.9));
#9950=CARTESIAN_POINT('Origin',(-4.8,0.,2.9));
#9951=CARTESIAN_POINT('',(-5.025,-2.75545529808154E-17,3.));
#9952=CARTESIAN_POINT('Origin',(-4.8,0.,3.));
#9953=CARTESIAN_POINT('',(-5.025,-2.75545529808154E-17,2.9));
#9954=CARTESIAN_POINT('Origin',(-4.8,-1.8,2.9));
#9955=CARTESIAN_POINT('',(-5.025,-1.8,3.));
#9956=CARTESIAN_POINT('Origin',(-4.8,-1.8,3.));
#9957=CARTESIAN_POINT('',(-5.025,-1.8,2.9));
#9958=CARTESIAN_POINT('Origin',(4.8,0.,2.9));
#9959=CARTESIAN_POINT('',(4.575,-2.75545529808154E-17,3.));
#9960=CARTESIAN_POINT('Origin',(4.8,0.,3.));
#9961=CARTESIAN_POINT('',(4.575,-2.75545529808154E-17,2.9));
#9962=CARTESIAN_POINT('Origin',(5.5,2.5,3.));
#9963=CARTESIAN_POINT('',(5.5,2.5,3.));
#9964=CARTESIAN_POINT('',(-5.5,2.5,3.));
#9965=CARTESIAN_POINT('',(5.5,2.5,3.));
#9966=CARTESIAN_POINT('',(-5.5,2.5,6.));
#9967=CARTESIAN_POINT('',(-5.5,2.5,3.));
#9968=CARTESIAN_POINT('',(5.5,2.5,6.));
#9969=CARTESIAN_POINT('',(5.5,2.5,6.));
#9970=CARTESIAN_POINT('',(5.5,2.5,3.));
#9971=CARTESIAN_POINT('Origin',(5.5,-2.5,3.));
#9972=CARTESIAN_POINT('',(5.5,-2.5,3.));
#9973=CARTESIAN_POINT('',(5.5,-2.5,3.));
#9974=CARTESIAN_POINT('',(5.5,-2.5,6.));
#9975=CARTESIAN_POINT('',(5.5,-2.5,6.));
#9976=CARTESIAN_POINT('',(5.5,-2.5,3.));
#9977=CARTESIAN_POINT('Origin',(-5.5,-2.5,3.));
#9978=CARTESIAN_POINT('',(-5.5,-2.5,3.));
#9979=CARTESIAN_POINT('',(-5.5,-2.5,3.));
#9980=CARTESIAN_POINT('',(-5.5,-2.5,6.));
#9981=CARTESIAN_POINT('',(-5.5,-2.5,6.));
#9982=CARTESIAN_POINT('',(-5.5,-2.5,3.));
#9983=CARTESIAN_POINT('Origin',(-5.5,2.5,3.));
#9984=CARTESIAN_POINT('',(-5.5,2.5,3.));
#9985=CARTESIAN_POINT('',(-5.5,2.5,6.));
#9986=CARTESIAN_POINT('Origin',(0.,0.,6.));
#9987=CARTESIAN_POINT('Origin',(0.,0.,3.));
#11359=UNCERTAINTY_MEASURE_WITH_UNIT(LENGTH_MEASURE(0.001),#11433,
'DISTANCE_ACCURACY_VALUE',
'Maximum model space distance between geometric entities at asserted c
onnectivities');
#11393=UNCERTAINTY_MEASURE_WITH_UNIT(LENGTH_MEASURE(0.001),#11433,
'DISTANCE_ACCURACY_VALUE',
'Maximum model space distance between geometric entities at asserted c
onnectivities');
#11398=(
GEOMETRIC_REPRESENTATION_CONTEXT(3)
GLOBAL_UNCERTAINTY_ASSIGNED_CONTEXT((#11359))
GLOBAL_UNIT_ASSIGNED_CONTEXT((#11433,#11435,#11436))
REPRESENTATION_CONTEXT('','3D')
);
#11432=(
GEOMETRIC_REPRESENTATION_CONTEXT(3)
GLOBAL_UNCERTAINTY_ASSIGNED_CONTEXT((#11393))
GLOBAL_UNIT_ASSIGNED_CONTEXT((#11433,#11435,#11436))
REPRESENTATION_CONTEXT('','3D')
);
#11433=(
LENGTH_UNIT()
NAMED_UNIT(*)
SI_UNIT(.CENTI.,.METRE.)
);
#11435=(
NAMED_UNIT(*)
PLANE_ANGLE_UNIT()
SI_UNIT($,.RADIAN.)
);
#11436=(
NAMED_UNIT(*)
SI_UNIT($,.STERADIAN.)
SOLID_ANGLE_UNIT()
);
#11441=SHAPE_DEFINITION_REPRESENTATION(#11479,#11567);
#11479=PRODUCT_DEFINITION_SHAPE('',$,#11606);
#11567=SHAPE_REPRESENTATION('',(#6572),#11398);
#11601=PRODUCT_DEFINITION_CONTEXT('part definition',#11717,'design');
#11606=PRODUCT_DEFINITION('Distributor','Distributor',#11644,
#11601);
#11644=PRODUCT_DEFINITION_FORMATION('',$,#11723);
#11717=APPLICATION_CONTEXT(
'Core Data for Automotive Mechanical Design Process');
#11718=PRODUCT_CONTEXT('part definition',#11717,'mechanical');
#11723=PRODUCT('Distributor','Distributor','Distributor',
(#11718));
#11827=COLOUR_RGB('Off White',0.89,0.88,0.83);
#11828=FILL_AREA_STYLE_COLOUR('',#11827);
#11829=FILL_AREA_STYLE('',(#11828));
#11830=SURFACE_STYLE_FILL_AREA(#11829);
#11831=SURFACE_SIDE_STYLE('',(#11830));
#11832=SURFACE_STYLE_USAGE(.BOTH.,#11831);
#11833=PRESENTATION_STYLE_ASSIGNMENT((#11832));
ENDSEC;
END-ISO-10303-21;
